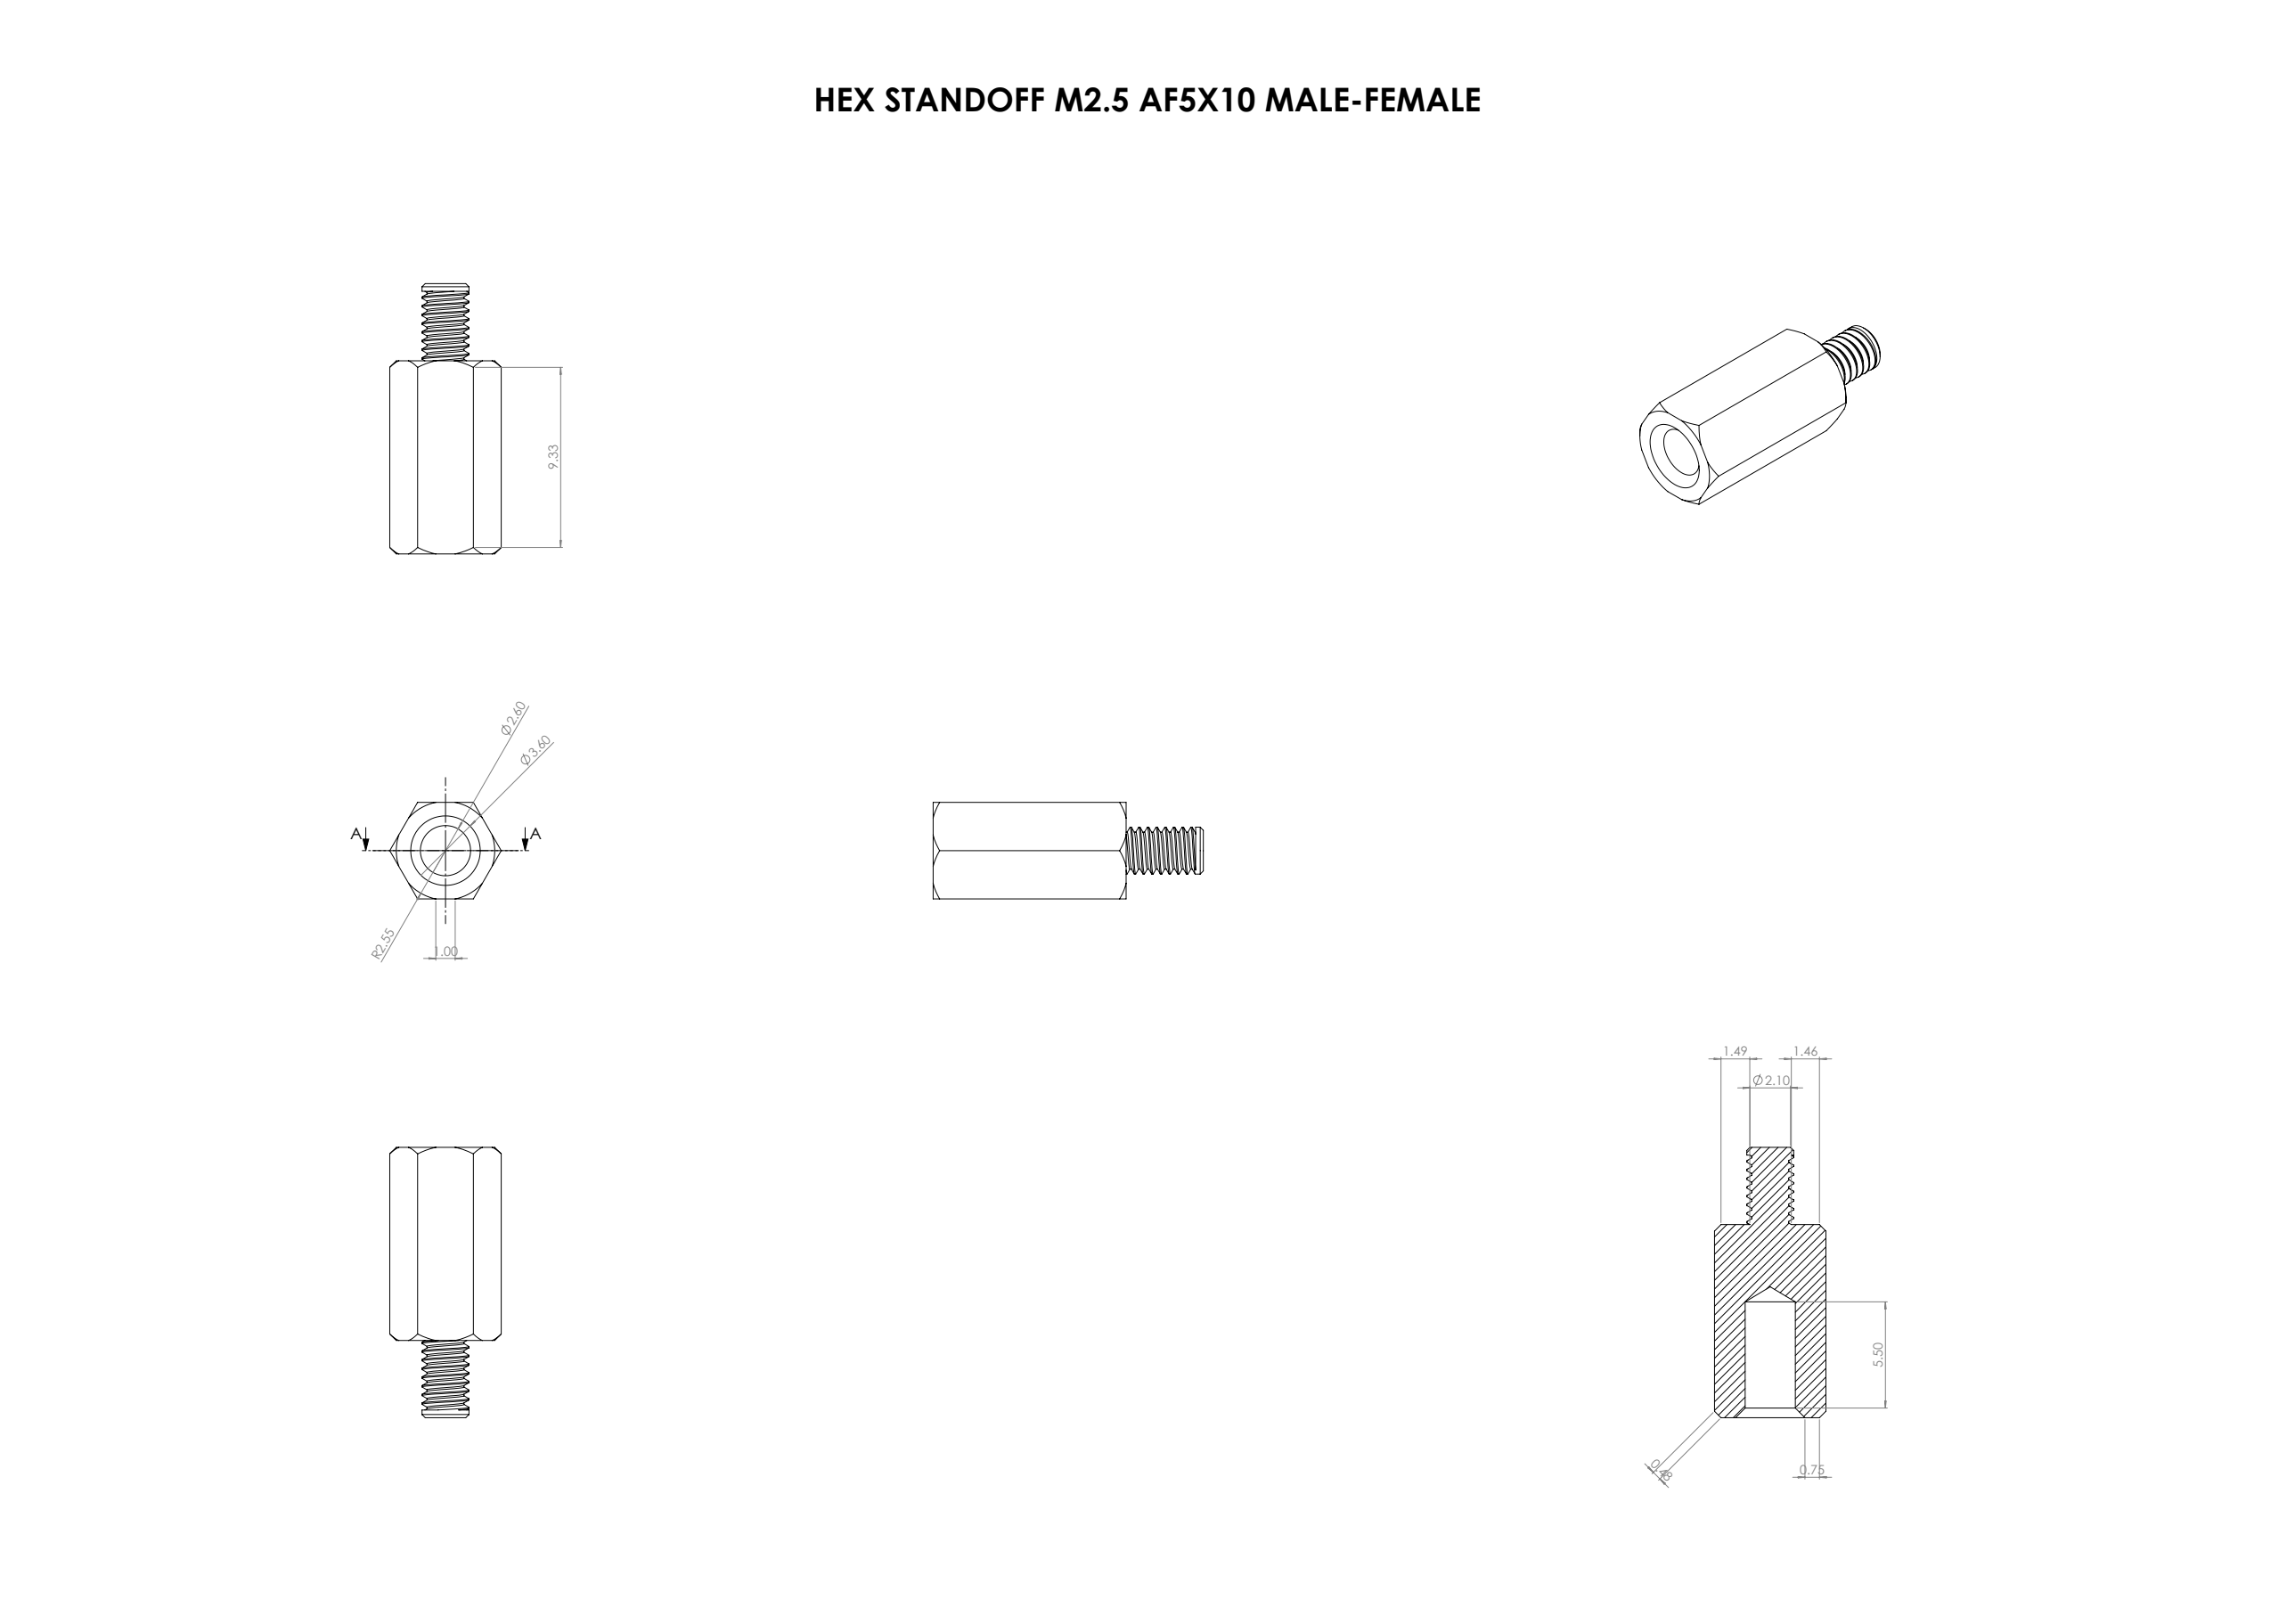
ISO-10303-21;
HEADER;
/* Generated by software containing ST-Developer
 * from STEP Tools, Inc. (www.steptools.com) 
 */

FILE_DESCRIPTION(
/* description */ (''),
/* implementation_level */ '2;1');

FILE_NAME(
/* name */ '14_Hex_Standoff_M2.5_AF5x10_Male-Female.step',
/* time_stamp */ '2026-10-19T23:00:43-07:00',
/* author */ (''),
/* organization */ (''),
/* preprocessor_version */ 'ST-DEVELOPER v20.2',
/* originating_system */ 'Autodesk Translation Framework v15.15.0.0',
/* authorisation */ '');

FILE_SCHEMA (('AUTOMOTIVE_DESIGN { 1 0 10303 214 3 1 1 }'));
ENDSEC;

DATA;
#10=MECHANICAL_DESIGN_GEOMETRIC_PRESENTATION_REPRESENTATION('',(#1010),#55002);
#227=(
BOUNDED_CURVE()
B_SPLINE_CURVE(2,(#39814,#39815,#39816),.UNSPECIFIED.,.F.,.F.)
B_SPLINE_CURVE_WITH_KNOTS((3,3),(0.0560176289802603,0.163687850794567),
 .UNSPECIFIED.)
CURVE()
GEOMETRIC_REPRESENTATION_ITEM()
RATIONAL_B_SPLINE_CURVE((1.01603499393247,1.02342774714042,1.))
REPRESENTATION_ITEM('')
);
#228=(
BOUNDED_CURVE()
B_SPLINE_CURVE(2,(#39818,#39819,#39820),.UNSPECIFIED.,.F.,.F.)
B_SPLINE_CURVE_WITH_KNOTS((3,3),(0.,0.107670221814307),.UNSPECIFIED.)
CURVE()
GEOMETRIC_REPRESENTATION_ITEM()
RATIONAL_B_SPLINE_CURVE((1.,1.02342774714043,1.01603499393248))
REPRESENTATION_ITEM('')
);
#229=(
BOUNDED_CURVE()
B_SPLINE_CURVE(2,(#39825,#39826,#39827),.UNSPECIFIED.,.F.,.F.)
B_SPLINE_CURVE_WITH_KNOTS((3,3),(0.0560176289802603,0.163687850794567),
 .UNSPECIFIED.)
CURVE()
GEOMETRIC_REPRESENTATION_ITEM()
RATIONAL_B_SPLINE_CURVE((1.01603499393248,1.02342774714042,1.))
REPRESENTATION_ITEM('')
);
#230=(
BOUNDED_CURVE()
B_SPLINE_CURVE(2,(#39829,#39830,#39831),.UNSPECIFIED.,.F.,.F.)
B_SPLINE_CURVE_WITH_KNOTS((3,3),(0.,0.107670221814307),.UNSPECIFIED.)
CURVE()
GEOMETRIC_REPRESENTATION_ITEM()
RATIONAL_B_SPLINE_CURVE((1.,1.02342774714042,1.01603499393248))
REPRESENTATION_ITEM('')
);
#231=(
BOUNDED_CURVE()
B_SPLINE_CURVE(2,(#39836,#39837,#39838),.UNSPECIFIED.,.F.,.F.)
B_SPLINE_CURVE_WITH_KNOTS((3,3),(0.0560176289802603,0.163687850794567),
 .UNSPECIFIED.)
CURVE()
GEOMETRIC_REPRESENTATION_ITEM()
RATIONAL_B_SPLINE_CURVE((1.01603499393248,1.02342774714042,1.))
REPRESENTATION_ITEM('')
);
#232=(
BOUNDED_CURVE()
B_SPLINE_CURVE(2,(#39840,#39841,#39842),.UNSPECIFIED.,.F.,.F.)
B_SPLINE_CURVE_WITH_KNOTS((3,3),(0.,0.107670221814307),.UNSPECIFIED.)
CURVE()
GEOMETRIC_REPRESENTATION_ITEM()
RATIONAL_B_SPLINE_CURVE((1.,1.02342774714043,1.01603499393248))
REPRESENTATION_ITEM('')
);
#233=(
BOUNDED_CURVE()
B_SPLINE_CURVE(2,(#39847,#39848,#39849),.UNSPECIFIED.,.F.,.F.)
B_SPLINE_CURVE_WITH_KNOTS((3,3),(0.0560176289802605,0.163687850794567),
 .UNSPECIFIED.)
CURVE()
GEOMETRIC_REPRESENTATION_ITEM()
RATIONAL_B_SPLINE_CURVE((1.01603499393247,1.02342774714041,1.))
REPRESENTATION_ITEM('')
);
#234=(
BOUNDED_CURVE()
B_SPLINE_CURVE(2,(#39851,#39852,#39853),.UNSPECIFIED.,.F.,.F.)
B_SPLINE_CURVE_WITH_KNOTS((3,3),(0.,0.107670221814307),.UNSPECIFIED.)
CURVE()
GEOMETRIC_REPRESENTATION_ITEM()
RATIONAL_B_SPLINE_CURVE((1.,1.02342774714042,1.01603499393247))
REPRESENTATION_ITEM('')
);
#235=(
BOUNDED_CURVE()
B_SPLINE_CURVE(2,(#39858,#39859,#39860),.UNSPECIFIED.,.F.,.F.)
B_SPLINE_CURVE_WITH_KNOTS((3,3),(0.0560176289802603,0.163687850794567),
 .UNSPECIFIED.)
CURVE()
GEOMETRIC_REPRESENTATION_ITEM()
RATIONAL_B_SPLINE_CURVE((1.01603499393247,1.02342774714041,1.))
REPRESENTATION_ITEM('')
);
#236=(
BOUNDED_CURVE()
B_SPLINE_CURVE(2,(#39862,#39863,#39864),.UNSPECIFIED.,.F.,.F.)
B_SPLINE_CURVE_WITH_KNOTS((3,3),(0.,0.107670221814307),.UNSPECIFIED.)
CURVE()
GEOMETRIC_REPRESENTATION_ITEM()
RATIONAL_B_SPLINE_CURVE((1.,1.02342774714042,1.01603499393247))
REPRESENTATION_ITEM('')
);
#237=(
BOUNDED_CURVE()
B_SPLINE_CURVE(2,(#39869,#39870,#39871),.UNSPECIFIED.,.F.,.F.)
B_SPLINE_CURVE_WITH_KNOTS((3,3),(0.,0.107670221814307),.UNSPECIFIED.)
CURVE()
GEOMETRIC_REPRESENTATION_ITEM()
RATIONAL_B_SPLINE_CURVE((1.,1.02342774714043,1.01603499393248))
REPRESENTATION_ITEM('')
);
#238=(
BOUNDED_CURVE()
B_SPLINE_CURVE(2,(#39874,#39875,#39876),.UNSPECIFIED.,.F.,.F.)
B_SPLINE_CURVE_WITH_KNOTS((3,3),(0.0560176289802603,0.163687850794567),
 .UNSPECIFIED.)
CURVE()
GEOMETRIC_REPRESENTATION_ITEM()
RATIONAL_B_SPLINE_CURVE((1.01603499393247,1.02342774714042,1.))
REPRESENTATION_ITEM('')
);
#239=(
BOUNDED_CURVE()
B_SPLINE_CURVE(2,(#39881,#39882,#39883),.UNSPECIFIED.,.F.,.F.)
B_SPLINE_CURVE_WITH_KNOTS((3,3),(0.0560176289802605,0.163687850794567),
 .UNSPECIFIED.)
CURVE()
GEOMETRIC_REPRESENTATION_ITEM()
RATIONAL_B_SPLINE_CURVE((1.01603499393247,1.02342774714041,1.))
REPRESENTATION_ITEM('')
);
#240=(
BOUNDED_CURVE()
B_SPLINE_CURVE(2,(#39887,#39888,#39889),.UNSPECIFIED.,.F.,.F.)
B_SPLINE_CURVE_WITH_KNOTS((3,3),(0.,0.107670221814307),.UNSPECIFIED.)
CURVE()
GEOMETRIC_REPRESENTATION_ITEM()
RATIONAL_B_SPLINE_CURVE((1.,1.02342774714041,1.01603499393247))
REPRESENTATION_ITEM('')
);
#241=(
BOUNDED_CURVE()
B_SPLINE_CURVE(2,(#39894,#39895,#39896),.UNSPECIFIED.,.F.,.F.)
B_SPLINE_CURVE_WITH_KNOTS((3,3),(0.0560176289802601,0.163687850794567),
 .UNSPECIFIED.)
CURVE()
GEOMETRIC_REPRESENTATION_ITEM()
RATIONAL_B_SPLINE_CURVE((1.01603499393247,1.02342774714041,1.))
REPRESENTATION_ITEM('')
);
#242=(
BOUNDED_CURVE()
B_SPLINE_CURVE(2,(#39900,#39901,#39902),.UNSPECIFIED.,.F.,.F.)
B_SPLINE_CURVE_WITH_KNOTS((3,3),(0.,0.107670221814307),.UNSPECIFIED.)
CURVE()
GEOMETRIC_REPRESENTATION_ITEM()
RATIONAL_B_SPLINE_CURVE((1.,1.02342774714041,1.01603499393247))
REPRESENTATION_ITEM('')
);
#243=(
BOUNDED_CURVE()
B_SPLINE_CURVE(2,(#39907,#39908,#39909),.UNSPECIFIED.,.F.,.F.)
B_SPLINE_CURVE_WITH_KNOTS((3,3),(0.0560176289802598,0.163687850794567),
 .UNSPECIFIED.)
CURVE()
GEOMETRIC_REPRESENTATION_ITEM()
RATIONAL_B_SPLINE_CURVE((1.01603499393248,1.02342774714042,1.))
REPRESENTATION_ITEM('')
);
#244=(
BOUNDED_CURVE()
B_SPLINE_CURVE(2,(#39913,#39914,#39915),.UNSPECIFIED.,.F.,.F.)
B_SPLINE_CURVE_WITH_KNOTS((3,3),(0.,0.107670221814307),.UNSPECIFIED.)
CURVE()
GEOMETRIC_REPRESENTATION_ITEM()
RATIONAL_B_SPLINE_CURVE((1.,1.02342774714041,1.01603499393247))
REPRESENTATION_ITEM('')
);
#245=(
BOUNDED_CURVE()
B_SPLINE_CURVE(2,(#39924,#39925,#39926),.UNSPECIFIED.,.F.,.F.)
B_SPLINE_CURVE_WITH_KNOTS((3,3),(0.0560176289802602,0.163687850794567),
 .UNSPECIFIED.)
CURVE()
GEOMETRIC_REPRESENTATION_ITEM()
RATIONAL_B_SPLINE_CURVE((1.01603499393248,1.02342774714042,1.))
REPRESENTATION_ITEM('')
);
#246=(
BOUNDED_CURVE()
B_SPLINE_CURVE(2,(#39930,#39931,#39932),.UNSPECIFIED.,.F.,.F.)
B_SPLINE_CURVE_WITH_KNOTS((3,3),(0.,0.107670221814307),.UNSPECIFIED.)
CURVE()
GEOMETRIC_REPRESENTATION_ITEM()
RATIONAL_B_SPLINE_CURVE((1.,1.02342774714041,1.01603499393247))
REPRESENTATION_ITEM('')
);
#247=(
BOUNDED_CURVE()
B_SPLINE_CURVE(2,(#39937,#39938,#39939),.UNSPECIFIED.,.F.,.F.)
B_SPLINE_CURVE_WITH_KNOTS((3,3),(0.,0.107670221814307),.UNSPECIFIED.)
CURVE()
GEOMETRIC_REPRESENTATION_ITEM()
RATIONAL_B_SPLINE_CURVE((1.,1.02342774714041,1.01603499393247))
REPRESENTATION_ITEM('')
);
#248=(
BOUNDED_CURVE()
B_SPLINE_CURVE(2,(#39942,#39943,#39944),.UNSPECIFIED.,.F.,.F.)
B_SPLINE_CURVE_WITH_KNOTS((3,3),(0.0560176289802595,0.163687850794568),
 .UNSPECIFIED.)
CURVE()
GEOMETRIC_REPRESENTATION_ITEM()
RATIONAL_B_SPLINE_CURVE((1.01603499393248,1.02342774714043,1.))
REPRESENTATION_ITEM('')
);
#249=(
BOUNDED_CURVE()
B_SPLINE_CURVE(2,(#39948,#39949,#39950),.UNSPECIFIED.,.F.,.F.)
B_SPLINE_CURVE_WITH_KNOTS((3,3),(0.05601762898026,0.163687850794567),
 .UNSPECIFIED.)
CURVE()
GEOMETRIC_REPRESENTATION_ITEM()
RATIONAL_B_SPLINE_CURVE((1.01603499393247,1.02342774714041,1.))
REPRESENTATION_ITEM('')
);
#250=(
BOUNDED_CURVE()
B_SPLINE_CURVE(2,(#39959,#39960,#39961),.UNSPECIFIED.,.F.,.F.)
B_SPLINE_CURVE_WITH_KNOTS((3,3),(0.,0.107670221814308),.UNSPECIFIED.)
CURVE()
GEOMETRIC_REPRESENTATION_ITEM()
RATIONAL_B_SPLINE_CURVE((1.,1.02342774714044,1.01603499393249))
REPRESENTATION_ITEM('')
);
#472=B_SPLINE_SURFACE_WITH_KNOTS('',3,3,((#39118,#39119,#39120,#39121,#39122,
#39123,#39124,#39125,#39126,#39127,#39128,#39129,#39130,#39131,#39132,#39133,
#39134,#39135,#39136,#39137,#39138,#39139,#39140,#39141,#39142,#39143,#39144,
#39145,#39146,#39147,#39148,#39149,#39150,#39151,#39152,#39153,#39154,#39155,
#39156,#39157,#39158,#39159,#39160,#39161,#39162,#39163,#39164,#39165,#39166,
#39167,#39168,#39169,#39170,#39171,#39172,#39173),(#39174,#39175,#39176,
#39177,#39178,#39179,#39180,#39181,#39182,#39183,#39184,#39185,#39186,#39187,
#39188,#39189,#39190,#39191,#39192,#39193,#39194,#39195,#39196,#39197,#39198,
#39199,#39200,#39201,#39202,#39203,#39204,#39205,#39206,#39207,#39208,#39209,
#39210,#39211,#39212,#39213,#39214,#39215,#39216,#39217,#39218,#39219,#39220,
#39221,#39222,#39223,#39224,#39225,#39226,#39227,#39228,#39229),(#39230,
#39231,#39232,#39233,#39234,#39235,#39236,#39237,#39238,#39239,#39240,#39241,
#39242,#39243,#39244,#39245,#39246,#39247,#39248,#39249,#39250,#39251,#39252,
#39253,#39254,#39255,#39256,#39257,#39258,#39259,#39260,#39261,#39262,#39263,
#39264,#39265,#39266,#39267,#39268,#39269,#39270,#39271,#39272,#39273,#39274,
#39275,#39276,#39277,#39278,#39279,#39280,#39281,#39282,#39283,#39284,#39285),
(#39286,#39287,#39288,#39289,#39290,#39291,#39292,#39293,#39294,#39295,
#39296,#39297,#39298,#39299,#39300,#39301,#39302,#39303,#39304,#39305,#39306,
#39307,#39308,#39309,#39310,#39311,#39312,#39313,#39314,#39315,#39316,#39317,
#39318,#39319,#39320,#39321,#39322,#39323,#39324,#39325,#39326,#39327,#39328,
#39329,#39330,#39331,#39332,#39333,#39334,#39335,#39336,#39337,#39338,#39339,
#39340,#39341)),.UNSPECIFIED.,.F.,.F.,.F.,(4,4),(4,1,1,1,1,1,1,1,1,1,1,
1,1,1,1,1,1,1,1,1,1,1,1,1,1,1,1,1,1,1,1,1,1,1,1,1,1,1,1,1,1,1,1,1,1,1,1,
1,1,1,1,1,1,4),(0.,0.0296469363228873),(11.5874873465742,12.5749444987495,
13.5624016509248,14.5498588031001,15.5373159552754,16.5247731074507,17.512230259626,
18.4996874118013,19.4871445639766,20.4746017161519,21.4620588683272,22.4495160205025,
23.4369731726778,24.4244303248531,25.4118874770284,26.3993446292037,27.386801781379,
28.3742589335543,29.3617160857296,30.3491732379048,31.3366303900801,32.3240875422554,
33.3115446944307,34.299001846606,35.2864589987813,36.2739161509566,37.2613733031319,
38.2488304553072,39.2362876074825,40.2237447596578,41.2112019118331,42.1986590640084,
43.1861162161837,44.173573368359,45.1610305205343,46.1484876727096,47.1359448248849,
48.1234019770602,49.1108591292355,50.0983162814107,51.085773433586,52.0732305857613,
53.0606877379366,54.0481448901119,55.0356020422872,56.0230591944625,57.0105163466378,
57.9979734988131,58.9854306509884,59.9728878031637,60.960344955339,61.9478021075143,
62.9352592596896,63.9227164118649),.UNSPECIFIED.);
#473=B_SPLINE_SURFACE_WITH_KNOTS('',3,3,((#39515,#39516,#39517,#39518,#39519,
#39520,#39521,#39522,#39523,#39524,#39525,#39526,#39527,#39528,#39529,#39530,
#39531,#39532,#39533,#39534,#39535,#39536,#39537,#39538,#39539,#39540,#39541,
#39542,#39543,#39544,#39545,#39546,#39547,#39548,#39549,#39550,#39551,#39552,
#39553,#39554,#39555,#39556,#39557,#39558,#39559,#39560,#39561,#39562,#39563,
#39564,#39565,#39566,#39567,#39568,#39569,#39570),(#39571,#39572,#39573,
#39574,#39575,#39576,#39577,#39578,#39579,#39580,#39581,#39582,#39583,#39584,
#39585,#39586,#39587,#39588,#39589,#39590,#39591,#39592,#39593,#39594,#39595,
#39596,#39597,#39598,#39599,#39600,#39601,#39602,#39603,#39604,#39605,#39606,
#39607,#39608,#39609,#39610,#39611,#39612,#39613,#39614,#39615,#39616,#39617,
#39618,#39619,#39620,#39621,#39622,#39623,#39624,#39625,#39626),(#39627,
#39628,#39629,#39630,#39631,#39632,#39633,#39634,#39635,#39636,#39637,#39638,
#39639,#39640,#39641,#39642,#39643,#39644,#39645,#39646,#39647,#39648,#39649,
#39650,#39651,#39652,#39653,#39654,#39655,#39656,#39657,#39658,#39659,#39660,
#39661,#39662,#39663,#39664,#39665,#39666,#39667,#39668,#39669,#39670,#39671,
#39672,#39673,#39674,#39675,#39676,#39677,#39678,#39679,#39680,#39681,#39682),
(#39683,#39684,#39685,#39686,#39687,#39688,#39689,#39690,#39691,#39692,
#39693,#39694,#39695,#39696,#39697,#39698,#39699,#39700,#39701,#39702,#39703,
#39704,#39705,#39706,#39707,#39708,#39709,#39710,#39711,#39712,#39713,#39714,
#39715,#39716,#39717,#39718,#39719,#39720,#39721,#39722,#39723,#39724,#39725,
#39726,#39727,#39728,#39729,#39730,#39731,#39732,#39733,#39734,#39735,#39736,
#39737,#39738)),.UNSPECIFIED.,.F.,.F.,.F.,(4,4),(4,1,1,1,1,1,1,1,1,1,1,
1,1,1,1,1,1,1,1,1,1,1,1,1,1,1,1,1,1,1,1,1,1,1,1,1,1,1,1,1,1,1,1,1,1,1,1,
1,1,1,1,1,1,4),(0.,0.0296469363228873),(14.896352608199,15.8838097603743,
16.8712669125496,17.8587240647249,18.8461812169001,19.8336383690754,20.8210955212507,
21.808552673426,22.7960098256013,23.7834669777766,24.7709241299519,25.7583812821272,
26.7458384343025,27.7332955864778,28.7207527386531,29.7082098908284,30.6956670430037,
31.683124195179,32.6705813473543,33.6580384995296,34.6454956517049,35.6329528038802,
36.6204099560555,37.6078671082307,38.595324260406,39.5827814125813,40.5702385647566,
41.5576957169319,42.5451528691072,43.5326100212825,44.5200671734578,45.5075243256331,
46.4949814778084,47.4824386299837,48.469895782159,49.4573529343343,50.4448100865096,
51.4322672386849,52.4197243908602,53.4071815430355,54.3946386952108,55.3820958473861,
56.3695529995614,57.3570101517367,58.3444673039119,59.3319244560872,60.3193816082625,
61.3068387604378,62.2942959126131,63.2817530647884,64.2692102169637,65.256667369139,
66.2441245213143,67.2315816734896),.UNSPECIFIED.);
#528=B_SPLINE_CURVE_WITH_KNOTS('',3,(#38534,#38535,#38536,#38537,#38538,
#38539,#38540,#38541,#38542,#38543,#38544,#38545,#38546,#38547,#38548,#38549,
#38550,#38551,#38552),.UNSPECIFIED.,.F.,.F.,(4,3,3,3,3,3,4),(-7.09479596692956,
-6.91220006522707,-5.92474291305177,-4.93728576087648,-3.94982860870118,
-2.96237145652589,-2.06974660785394),.UNSPECIFIED.);
#529=B_SPLINE_CURVE_WITH_KNOTS('',3,(#38560,#38561,#38562,#38563,#38564,
#38565,#38566,#38567,#38568,#38569,#38570,#38571,#38572,#38573,#38574,#38575),
 .UNSPECIFIED.,.F.,.F.,(4,3,3,3,3,4),(0.,0.987457152175289,1.97491430435059,
2.96237145652588,3.94982860870118,4.12047592137467),.UNSPECIFIED.);
#530=B_SPLINE_CURVE_WITH_KNOTS('',3,(#38580,#38581,#38582,#38583,#38584,
#38585,#38586,#38587,#38588,#38589,#38590,#38591,#38592,#38593,#38594,#38595,
#38596,#38597,#38598,#38599,#38600,#38601),.UNSPECIFIED.,.F.,.F.,(4,3,3,
3,3,3,3,4),(-13.3779812741091,-12.8369429782788,-11.8494858261035,-10.8620286739282,
-9.87457152175295,-8.88711436957765,-7.89965721740236,-7.09479596692956),
 .UNSPECIFIED.);
#531=B_SPLINE_CURVE_WITH_KNOTS('',3,(#38602,#38603,#38604,#38605,#38606,
#38607,#38608,#38609,#38610,#38611,#38612,#38613,#38614,#38615,#38616,#38617,
#38618,#38619,#38620,#38621,#38622,#38623),.UNSPECIFIED.,.F.,.F.,(4,3,3,
3,3,3,3,4),(4.12047592137467,4.93728576087648,5.92474291305177,6.91220006522707,
7.89965721740236,8.88711436957765,9.87457152175295,10.4036612285542),
 .UNSPECIFIED.);
#532=B_SPLINE_CURVE_WITH_KNOTS('',3,(#38628,#38629,#38630,#38631,#38632,
#38633,#38634,#38635,#38636,#38637,#38638,#38639,#38640,#38641,#38642,#38643,
#38644,#38645,#38646,#38647,#38648,#38649),.UNSPECIFIED.,.F.,.F.,(4,3,3,
3,3,3,3,4),(-19.6611665812887,-18.7616858913306,-17.7742287391553,-16.78677158698,
-15.7993144348047,-14.8118572826294,-13.8244001304541,-13.3779812741091),
 .UNSPECIFIED.);
#533=B_SPLINE_CURVE_WITH_KNOTS('',3,(#38650,#38651,#38652,#38653,#38654,
#38655,#38656,#38657,#38658,#38659,#38660,#38661,#38662,#38663,#38664,#38665,
#38666,#38667,#38668,#38669,#38670,#38671),.UNSPECIFIED.,.F.,.F.,(4,3,3,
3,3,3,3,4),(10.4036612285542,10.8620286739282,11.8494858261035,12.8369429782788,
13.8244001304541,14.8118572826294,15.7993144348047,16.6868465357338),
 .UNSPECIFIED.);
#534=B_SPLINE_CURVE_WITH_KNOTS('',3,(#38676,#38677,#38678,#38679,#38680,
#38681,#38682,#38683,#38684,#38685,#38686,#38687,#38688,#38689,#38690,#38691,
#38692,#38693,#38694,#38695,#38696,#38697,#38698,#38699,#38700),
 .UNSPECIFIED.,.F.,.F.,(4,3,3,3,3,3,3,3,4),(-25.9443518884683,-25.6738859565577,
-24.6864288043824,-23.6989716522071,-22.7115145000318,-21.7240573478565,
-20.7366001956812,-19.7491430435059,-19.6611665812887),.UNSPECIFIED.);
#535=B_SPLINE_CURVE_WITH_KNOTS('',3,(#38701,#38702,#38703,#38704,#38705,
#38706,#38707,#38708,#38709,#38710,#38711,#38712,#38713,#38714,#38715,#38716,
#38717,#38718,#38719,#38720,#38721,#38722,#38723,#38724,#38725),
 .UNSPECIFIED.,.F.,.F.,(4,3,3,3,3,3,3,3,4),(16.6868465357338,16.78677158698,
17.7742287391553,18.7616858913306,19.7491430435059,20.7366001956812,21.7240573478565,
22.7115145000318,22.9700318429134),.UNSPECIFIED.);
#536=B_SPLINE_CURVE_WITH_KNOTS('',3,(#38730,#38731,#38732,#38733,#38734,
#38735,#38736,#38737,#38738,#38739,#38740,#38741,#38742,#38743,#38744,#38745,
#38746,#38747,#38748,#38749,#38750,#38751),.UNSPECIFIED.,.F.,.F.,(4,3,3,
3,3,3,3,4),(-32.2275371956479,-31.5986288696094,-30.6111717174341,-29.6237145652589,
-28.6362574130836,-27.6488002609083,-26.661343108733,-25.9443518884683),
 .UNSPECIFIED.);
#537=B_SPLINE_CURVE_WITH_KNOTS('',3,(#38752,#38753,#38754,#38755,#38756,
#38757,#38758,#38759,#38760,#38761,#38762,#38763,#38764,#38765,#38766,#38767,
#38768,#38769,#38770,#38771,#38772,#38773),.UNSPECIFIED.,.F.,.F.,(4,3,3,
3,3,3,3,4),(22.9700318429134,23.6989716522071,24.6864288043824,25.6738859565577,
26.661343108733,27.6488002609083,28.6362574130836,29.253217150093),
 .UNSPECIFIED.);
#538=B_SPLINE_CURVE_WITH_KNOTS('',3,(#38778,#38779,#38780,#38781,#38782,
#38783,#38784,#38785,#38786,#38787,#38788,#38789,#38790,#38791,#38792,#38793,
#38794,#38795,#38796,#38797,#38798,#38799),.UNSPECIFIED.,.F.,.F.,(4,3,3,
3,3,3,3,4),(-38.5107225028275,-37.5233717826612,-36.5359146304859,-35.5484574783106,
-34.5610003261353,-33.57354317396,-32.5860860217847,-32.2275371956479),
 .UNSPECIFIED.);
#539=B_SPLINE_CURVE_WITH_KNOTS('',3,(#38800,#38801,#38802,#38803,#38804,
#38805,#38806,#38807,#38808,#38809,#38810,#38811,#38812,#38813,#38814,#38815,
#38816,#38817,#38818,#38819,#38820,#38821),.UNSPECIFIED.,.F.,.F.,(4,3,3,
3,3,3,3,4),(29.253217150093,29.6237145652588,30.6111717174341,31.5986288696094,
32.5860860217847,33.57354317396,34.5610003261353,35.5364024572726),
 .UNSPECIFIED.);
#540=B_SPLINE_CURVE_WITH_KNOTS('',3,(#38826,#38827,#38828,#38829,#38830,
#38831,#38832,#38833,#38834,#38835,#38836,#38837,#38838,#38839,#38840,#38841,
#38842,#38843,#38844,#38845,#38846,#38847),.UNSPECIFIED.,.F.,.F.,(4,3,3,
3,3,3,3,4),(-44.7939078100071,-44.4355718478883,-43.448114695713,-42.4606575435377,
-41.4732003913624,-40.4857432391871,-39.4982860870118,-38.5107225028275),
 .UNSPECIFIED.);
#541=B_SPLINE_CURVE_WITH_KNOTS('',3,(#38848,#38849,#38850,#38851,#38852,
#38853,#38854,#38855,#38856,#38857,#38858,#38859,#38860,#38861,#38862,#38863,
#38864,#38865,#38866,#38867,#38868,#38869,#38870,#38871,#38872),
 .UNSPECIFIED.,.F.,.F.,(4,3,3,3,3,3,3,3,4),(35.5364024572726,35.5484574783106,
36.5359146304859,37.5233717826612,38.5108289348365,39.4982860870118,40.4857432391871,
41.4732003913624,41.8195877644522),.UNSPECIFIED.);
#542=B_SPLINE_CURVE_WITH_KNOTS('',3,(#38877,#38878,#38879,#38880,#38881,
#38882,#38883,#38884,#38885,#38886,#38887,#38888,#38889,#38890,#38891,#38892,
#38893,#38894,#38895,#38896,#38897,#38898),.UNSPECIFIED.,.F.,.F.,(4,3,3,
3,3,3,3,4),(-51.0770931171867,-50.36031476094,-49.3728576087648,-48.3854004565895,
-47.3979433044142,-46.4104861522389,-45.4230290000636,-44.7939078100071),
 .UNSPECIFIED.);
#543=B_SPLINE_CURVE_WITH_KNOTS('',3,(#38899,#38900,#38901,#38902,#38903,
#38904,#38905,#38906,#38907,#38908,#38909,#38910,#38911,#38912,#38913,#38914,
#38915,#38916,#38917,#38918,#38919,#38920),.UNSPECIFIED.,.F.,.F.,(4,3,3,
3,3,3,3,4),(41.8195877644522,42.4606575435377,43.448114695713,44.4355718478883,
45.4230290000636,46.4104861522389,47.3979433044142,48.1027730716318),
 .UNSPECIFIED.);
#544=B_SPLINE_CURVE_WITH_KNOTS('',3,(#38926,#38927,#38928,#38929,#38930,
#38931,#38932,#38933,#38934),.UNSPECIFIED.,.F.,.F.,(4,1,1,1,1,1,4),(59.6902604182061,
60.3193816082625,61.3068387604378,62.2942959126131,63.2817530647884,64.2692102169637,
65.1618350656357),.UNSPECIFIED.);
#545=B_SPLINE_CURVE_WITH_KNOTS('',3,(#38937,#38938,#38939,#38940,#38941,
#38942,#38943,#38944),.UNSPECIFIED.,.F.,.F.,(4,1,1,1,1,4),(59.6902604182061,
59.9728878031637,60.960344955339,61.9478021075143,62.9352592596896,63.9227164118649),
 .UNSPECIFIED.);
#546=B_SPLINE_CURVE_WITH_KNOTS('',3,(#38949,#38950,#38951,#38952,#38953,
#38954,#38955,#38956,#38957,#38958,#38959),.UNSPECIFIED.,.F.,.F.,(4,1,1,
1,1,1,1,1,4),(53.4070751110265,53.4071815430355,54.3946386952108,55.3820958473861,
56.3695529995614,57.3570101517367,58.3444673039119,59.3319244560872,59.6902604182061),
 .UNSPECIFIED.);
#547=B_SPLINE_CURVE_WITH_KNOTS('',3,(#38960,#38961,#38962,#38963,#38964,
#38965,#38966,#38967,#38968,#38969),.UNSPECIFIED.,.F.,.F.,(4,1,1,1,1,1,
1,4),(53.4070751110265,54.0481448901119,55.0356020422872,56.0230591944625,
57.0105163466378,57.9979734988131,58.9854306509884,59.6902604182061),
 .UNSPECIFIED.);
#548=B_SPLINE_CURVE_WITH_KNOTS('',3,(#38974,#38975,#38976,#38977,#38978,
#38979,#38980,#38981,#38982,#38983),.UNSPECIFIED.,.F.,.F.,(4,1,1,1,1,1,
1,4),(47.1238898038469,47.4824386299837,48.469895782159,49.4573529343343,
50.4448100865096,51.4322672386849,52.4197243908602,53.4070751110265),
 .UNSPECIFIED.);
#549=B_SPLINE_CURVE_WITH_KNOTS('',3,(#38984,#38985,#38986,#38987,#38988,
#38989,#38990,#38991,#38992,#38993,#38994),.UNSPECIFIED.,.F.,.F.,(4,1,1,
1,1,1,1,1,4),(47.1238898038469,47.1359448248849,48.1234019770602,49.1108591292355,
50.0983162814107,51.085773433586,52.0732305857613,53.0606877379366,53.4070751110265),
 .UNSPECIFIED.);
#550=B_SPLINE_CURVE_WITH_KNOTS('',3,(#38999,#39000,#39001,#39002,#39003,
#39004,#39005,#39006,#39007,#39008),.UNSPECIFIED.,.F.,.F.,(4,1,1,1,1,1,
1,4),(40.8407044966673,41.5576957169319,42.5451528691072,43.5326100212825,
44.5200671734578,45.5075243256331,46.4949814778084,47.1238898038469),
 .UNSPECIFIED.);
#551=B_SPLINE_CURVE_WITH_KNOTS('',3,(#39009,#39010,#39011,#39012,#39013,
#39014,#39015,#39016,#39017,#39018),.UNSPECIFIED.,.F.,.F.,(4,1,1,1,1,1,
1,4),(40.8407044966673,41.2112019118331,42.1986590640084,43.1861162161837,
44.173573368359,45.1610305205343,46.1484876727096,47.1238898038469),
 .UNSPECIFIED.);
#552=B_SPLINE_CURVE_WITH_KNOTS('',3,(#39023,#39024,#39025,#39026,#39027,
#39028,#39029,#39030,#39031,#39032,#39033),.UNSPECIFIED.,.F.,.F.,(4,1,1,
1,1,1,1,1,4),(34.5575191894877,34.6454956517049,35.6329528038802,36.6204099560555,
37.6078671082307,38.595324260406,39.5827814125813,40.5702385647566,40.8407044966673),
 .UNSPECIFIED.);
#553=B_SPLINE_CURVE_WITH_KNOTS('',3,(#39034,#39035,#39036,#39037,#39038,
#39039,#39040,#39041,#39042,#39043),.UNSPECIFIED.,.F.,.F.,(4,1,1,1,1,1,
1,4),(34.5575191894877,35.2864589987813,36.2739161509566,37.2613733031319,
38.2488304553072,39.2362876074825,40.2237447596578,40.8407044966673),
 .UNSPECIFIED.);
#554=B_SPLINE_CURVE_WITH_KNOTS('',3,(#39048,#39049,#39050,#39051,#39052,
#39053,#39054,#39055,#39056,#39057),.UNSPECIFIED.,.F.,.F.,(4,1,1,1,1,1,
1,4),(28.2743338823081,28.7207527386531,29.7082098908284,30.6956670430037,
31.683124195179,32.6705813473543,33.6580384995296,34.5575191894877),
 .UNSPECIFIED.);
#555=B_SPLINE_CURVE_WITH_KNOTS('',3,(#39058,#39059,#39060,#39061,#39062,
#39063,#39064,#39065,#39066,#39067,#39068),.UNSPECIFIED.,.F.,.F.,(4,1,1,
1,1,1,1,1,4),(28.2743338823081,28.3742589335543,29.3617160857296,30.3491732379048,
31.3366303900801,32.3240875422554,33.3115446944307,34.299001846606,34.5575191894877),
 .UNSPECIFIED.);
#556=B_SPLINE_CURVE_WITH_KNOTS('',3,(#39073,#39074,#39075,#39076,#39077,
#39078,#39079,#39080,#39081,#39082),.UNSPECIFIED.,.F.,.F.,(4,1,1,1,1,1,
1,4),(21.9911485751285,22.7960098256013,23.7834669777766,24.7709241299519,
25.7583812821272,26.7458384343025,27.7332955864778,28.2743338823081),
 .UNSPECIFIED.);
#557=B_SPLINE_CURVE_WITH_KNOTS('',3,(#39083,#39084,#39085,#39086,#39087,
#39088,#39089,#39090,#39091,#39092),.UNSPECIFIED.,.F.,.F.,(4,1,1,1,1,1,
1,4),(21.9911485751285,22.4495160205025,23.4369731726778,24.4244303248531,
25.4118874770284,26.3993446292037,27.386801781379,28.2743338823081),
 .UNSPECIFIED.);
#558=B_SPLINE_CURVE_WITH_KNOTS('',3,(#39097,#39098,#39099,#39100,#39101,
#39102,#39103,#39104,#39105,#39106,#39107),.UNSPECIFIED.,.F.,.F.,(4,1,1,
1,1,1,1,1,4),(15.7079632679489,15.8838097603743,16.8712669125496,17.8587240647249,
18.8461812169001,19.8336383690754,20.8210955212507,21.808552673426,21.9911485751285),
 .UNSPECIFIED.);
#559=B_SPLINE_CURVE_WITH_KNOTS('',3,(#39108,#39109,#39110,#39111,#39112,
#39113,#39114,#39115,#39116,#39117),.UNSPECIFIED.,.F.,.F.,(4,1,1,1,1,1,
1,4),(15.7079632679489,16.5247731074507,17.512230259626,18.4996874118013,
19.4871445639766,20.4746017161519,21.4620588683272,21.9911485751285),
 .UNSPECIFIED.);
#560=B_SPLINE_CURVE_WITH_KNOTS('',3,(#39343,#39344,#39345,#39346,#39347,
#39348,#39349,#39350,#39351,#39352,#39353,#39354,#39355,#39356,#39357,#39358,
#39359,#39360,#39361,#39362,#39363,#39364,#39365,#39366,#39367,#39368,#39369,
#39370,#39371,#39372,#39373,#39374,#39375,#39376,#39377,#39378,#39379,#39380,
#39381,#39382,#39383,#39384,#39385,#39386,#39387,#39388,#39389,#39390,#39391),
 .UNSPECIFIED.,.F.,.F.,(4,3,3,3,3,3,3,3,3,3,3,3,3,3,3,3,4),(-0.226379821609611,
-0.214890180424997,-0.195063355378614,-0.183728168968286,-0.169237877031892,
-0.156768292348793,-0.131336338642949,-0.121264777035684,-0.11376486268334,
-0.101603376860372,-0.0859957740860565,-0.07722199741945,-0.0531920110136073,
-0.041845954216628,-0.0323163699760562,-0.00989131159632156,0.),
 .UNSPECIFIED.);
#561=B_SPLINE_CURVE_WITH_KNOTS('',3,(#39392,#39393,#39394,#39395,#39396,
#39397,#39398,#39399,#39400,#39401),.UNSPECIFIED.,.F.,.F.,(4,3,3,4),(48.1027730716318,
48.3854004565894,49.3728576087647,50.2654824574367),.UNSPECIFIED.);
#562=B_SPLINE_CURVE_WITH_KNOTS('',3,(#39403,#39404,#39405,#39406,#39407,
#39408,#39409,#39410,#39411,#39412,#39413,#39414,#39415,#39416,#39417,#39418,
#39419,#39420,#39421,#39422,#39423,#39424,#39425,#39426,#39427,#39428,#39429,
#39430,#39431,#39432,#39433,#39434,#39435,#39436,#39437,#39438,#39439,#39440,
#39441,#39442,#39443,#39444,#39445,#39446,#39447,#39448,#39449,#39450,#39451),
 .UNSPECIFIED.,.F.,.F.,(4,3,3,3,3,3,3,3,3,3,3,3,3,3,3,3,4),(-0.227523845437318,
-0.218254285946759,-0.205376019353374,-0.194839584423376,-0.181726252813619,
-0.172870003901879,-0.148477559368614,-0.136842916469509,-0.12791553259114,
-0.115084966565271,-0.0973336680873777,-0.0847825202648984,-0.0635868901986738,
-0.0502811887773191,-0.0410407821760877,-0.014115200632659,0.),
 .UNSPECIFIED.);
#563=B_SPLINE_CURVE_WITH_KNOTS('',3,(#39452,#39453,#39454,#39455,#39456,
#39457),.UNSPECIFIED.,.F.,.F.,(4,1,1,4),(13.6572339544282,14.5498588031001,
15.5373159552754,15.7079632679489),.UNSPECIFIED.);
#564=B_SPLINE_CURVE_WITH_KNOTS('',3,(#39460,#39461,#39462,#39463,#39464,
#39465,#39466,#39467,#39468,#39469,#39470,#39471,#39472,#39473,#39474,#39475,
#39476,#39477,#39478,#39479,#39480,#39481,#39482,#39483,#39484,#39485,#39486,
#39487,#39488,#39489,#39490,#39491,#39492,#39493,#39494,#39495,#39496,#39497,
#39498,#39499,#39500,#39501,#39502,#39503,#39504,#39505,#39506,#39507,#39508),
 .UNSPECIFIED.,.F.,.F.,(4,3,3,3,3,3,3,3,3,3,3,3,3,3,3,3,4),(-0.226379821609596,
-0.214890180424979,-0.195063350039947,-0.183728164322639,-0.169237850825561,
-0.156768290223532,-0.131336328824517,-0.12126472687929,-0.113764786721133,
-0.101603376860369,-0.0859957671104269,-0.0772219948002901,-0.0531920146182027,
-0.0418459669675516,-0.0323163753079122,-0.00989133560397837,0.),
 .UNSPECIFIED.);
#565=B_SPLINE_CURVE_WITH_KNOTS('',3,(#39511,#39512,#39513,#39514),
 .UNSPECIFIED.,.F.,.F.,(4,4),(14.896352608199,15.7079632679489),
 .UNSPECIFIED.);
#566=B_SPLINE_CURVE_WITH_KNOTS('',3,(#39740,#39741,#39742,#39743,#39744,
#39745,#39746,#39747,#39748,#39749,#39750,#39751,#39752,#39753,#39754,#39755,
#39756,#39757,#39758,#39759,#39760,#39761,#39762,#39763,#39764,#39765,#39766,
#39767,#39768,#39769,#39770,#39771,#39772,#39773,#39774,#39775,#39776,#39777,
#39778,#39779,#39780,#39781,#39782,#39783,#39784,#39785,#39786,#39787,#39788),
 .UNSPECIFIED.,.F.,.F.,(4,3,3,3,3,3,3,3,3,3,3,3,3,3,3,3,4),(-0.227523845437314,
-0.218254285946756,-0.205376031384273,-0.194839581377744,-0.181726328485879,
-0.172870086995034,-0.148477642599549,-0.13684302479023,-0.127915530672829,
-0.11508496656527,-0.0973336777498854,-0.0847825188673741,-0.0635868891505306,
-0.050281187305254,-0.0410407836210242,-0.0141152073468077,0.),
 .UNSPECIFIED.);
#567=B_SPLINE_CURVE_WITH_KNOTS('',3,(#39789,#39790,#39791,#39792,#39793,
#39794,#39795),.UNSPECIFIED.,.F.,.F.,(4,3,4),(-52.3352290652906,-51.3477719131153,
-51.0770931171867),.UNSPECIFIED.);
#970=SHAPE_REPRESENTATION_RELATIONSHIP('SRR','None',#55118,#990);
#990=ADVANCED_BREP_SHAPE_REPRESENTATION('',(#1030),#54996);
#1010=STYLED_ITEM('',(#55379),#1030);
#1030=MANIFOLD_SOLID_BREP('Hex Standoff',#24543);
#1261=FACE_BOUND('',#4742,.T.);
#1262=FACE_BOUND('',#4755,.T.);
#1548=PLANE('',#26206);
#1549=PLANE('',#26229);
#1550=PLANE('',#26230);
#1551=PLANE('',#26231);
#1552=PLANE('',#26232);
#1553=PLANE('',#26233);
#1554=PLANE('',#26246);
#1555=PLANE('',#26247);
#1556=PLANE('',#26250);
#1557=PLANE('',#26251);
#2202=CYLINDRICAL_SURFACE('',#26186,0.1215);
#2203=CYLINDRICAL_SURFACE('',#26190,0.1215);
#2204=CYLINDRICAL_SURFACE('',#26191,0.1215);
#2205=CYLINDRICAL_SURFACE('',#26192,0.1215);
#2206=CYLINDRICAL_SURFACE('',#26193,0.1215);
#2207=CYLINDRICAL_SURFACE('',#26194,0.1215);
#2208=CYLINDRICAL_SURFACE('',#26195,0.1215);
#2209=CYLINDRICAL_SURFACE('',#26196,0.1215);
#2210=CYLINDRICAL_SURFACE('',#26197,0.095825);
#2211=CYLINDRICAL_SURFACE('',#26199,0.095825);
#2212=CYLINDRICAL_SURFACE('',#26200,0.095825);
#2213=CYLINDRICAL_SURFACE('',#26201,0.095825);
#2214=CYLINDRICAL_SURFACE('',#26202,0.095825);
#2215=CYLINDRICAL_SURFACE('',#26203,0.095825);
#2216=CYLINDRICAL_SURFACE('',#26204,0.095825);
#2217=CYLINDRICAL_SURFACE('',#26205,0.095825);
#2218=CYLINDRICAL_SURFACE('',#26208,0.095825);
#2219=CYLINDRICAL_SURFACE('',#26209,0.1215);
#2220=CYLINDRICAL_SURFACE('',#26213,0.13);
#3119=FACE_OUTER_BOUND('',#4708,.T.);
#3120=FACE_OUTER_BOUND('',#4709,.T.);
#3121=FACE_OUTER_BOUND('',#4710,.T.);
#3122=FACE_OUTER_BOUND('',#4711,.T.);
#3123=FACE_OUTER_BOUND('',#4712,.T.);
#3124=FACE_OUTER_BOUND('',#4713,.T.);
#3125=FACE_OUTER_BOUND('',#4714,.T.);
#3126=FACE_OUTER_BOUND('',#4715,.T.);
#3127=FACE_OUTER_BOUND('',#4716,.T.);
#3128=FACE_OUTER_BOUND('',#4717,.T.);
#3129=FACE_OUTER_BOUND('',#4718,.T.);
#3130=FACE_OUTER_BOUND('',#4719,.T.);
#3131=FACE_OUTER_BOUND('',#4720,.T.);
#3132=FACE_OUTER_BOUND('',#4721,.T.);
#3133=FACE_OUTER_BOUND('',#4722,.T.);
#3134=FACE_OUTER_BOUND('',#4723,.T.);
#3135=FACE_OUTER_BOUND('',#4724,.T.);
#3136=FACE_OUTER_BOUND('',#4725,.T.);
#3137=FACE_OUTER_BOUND('',#4726,.T.);
#3138=FACE_OUTER_BOUND('',#4727,.T.);
#3139=FACE_OUTER_BOUND('',#4728,.T.);
#3140=FACE_OUTER_BOUND('',#4729,.T.);
#3141=FACE_OUTER_BOUND('',#4730,.T.);
#3142=FACE_OUTER_BOUND('',#4731,.T.);
#3143=FACE_OUTER_BOUND('',#4732,.T.);
#3144=FACE_OUTER_BOUND('',#4733,.T.);
#3145=FACE_OUTER_BOUND('',#4734,.T.);
#3146=FACE_OUTER_BOUND('',#4735,.T.);
#3147=FACE_OUTER_BOUND('',#4736,.T.);
#3148=FACE_OUTER_BOUND('',#4737,.T.);
#3149=FACE_OUTER_BOUND('',#4738,.T.);
#3150=FACE_OUTER_BOUND('',#4739,.T.);
#3151=FACE_OUTER_BOUND('',#4740,.T.);
#3152=FACE_OUTER_BOUND('',#4741,.T.);
#3153=FACE_OUTER_BOUND('',#4743,.T.);
#3154=FACE_OUTER_BOUND('',#4744,.T.);
#3155=FACE_OUTER_BOUND('',#4745,.T.);
#3156=FACE_OUTER_BOUND('',#4746,.T.);
#3157=FACE_OUTER_BOUND('',#4747,.T.);
#3158=FACE_OUTER_BOUND('',#4748,.T.);
#3159=FACE_OUTER_BOUND('',#4749,.T.);
#3160=FACE_OUTER_BOUND('',#4750,.T.);
#3161=FACE_OUTER_BOUND('',#4751,.T.);
#3162=FACE_OUTER_BOUND('',#4752,.T.);
#3163=FACE_OUTER_BOUND('',#4753,.T.);
#3164=FACE_OUTER_BOUND('',#4754,.T.);
#4708=EDGE_LOOP('',(#19198,#19199,#19200,#19201,#19202,#19203,#19204,#19205));
#4709=EDGE_LOOP('',(#19206,#19207,#19208,#19209));
#4710=EDGE_LOOP('',(#19210,#19211,#19212,#19213));
#4711=EDGE_LOOP('',(#19214,#19215,#19216,#19217));
#4712=EDGE_LOOP('',(#19218,#19219,#19220,#19221));
#4713=EDGE_LOOP('',(#19222,#19223,#19224,#19225));
#4714=EDGE_LOOP('',(#19226,#19227,#19228,#19229));
#4715=EDGE_LOOP('',(#19230,#19231,#19232,#19233));
#4716=EDGE_LOOP('',(#19234,#19235,#19236,#19237));
#4717=EDGE_LOOP('',(#19238,#19239,#19240,#19241));
#4718=EDGE_LOOP('',(#19242,#19243,#19244,#19245));
#4719=EDGE_LOOP('',(#19246,#19247,#19248,#19249));
#4720=EDGE_LOOP('',(#19250,#19251,#19252,#19253));
#4721=EDGE_LOOP('',(#19254,#19255,#19256,#19257));
#4722=EDGE_LOOP('',(#19258,#19259,#19260,#19261));
#4723=EDGE_LOOP('',(#19262,#19263,#19264,#19265));
#4724=EDGE_LOOP('',(#19266,#19267,#19268,#19269,#19270,#19271,#19272,#19273,
#19274,#19275,#19276,#19277,#19278,#19279,#19280,#19281,#19282,#19283,#19284,
#19285));
#4725=EDGE_LOOP('',(#19286,#19287,#19288,#19289,#19290));
#4726=EDGE_LOOP('',(#19291,#19292,#19293,#19294));
#4727=EDGE_LOOP('',(#19295,#19296,#19297,#19298,#19299,#19300,#19301,#19302,
#19303,#19304,#19305,#19306,#19307,#19308,#19309,#19310,#19311,#19312,#19313,
#19314));
#4728=EDGE_LOOP('',(#19315,#19316,#19317,#19318));
#4729=EDGE_LOOP('',(#19319,#19320,#19321));
#4730=EDGE_LOOP('',(#19322,#19323,#19324,#19325));
#4731=EDGE_LOOP('',(#19326,#19327,#19328,#19329));
#4732=EDGE_LOOP('',(#19330,#19331,#19332));
#4733=EDGE_LOOP('',(#19333,#19334,#19335));
#4734=EDGE_LOOP('',(#19336,#19337,#19338));
#4735=EDGE_LOOP('',(#19339,#19340,#19341));
#4736=EDGE_LOOP('',(#19342,#19343,#19344));
#4737=EDGE_LOOP('',(#19345,#19346,#19347));
#4738=EDGE_LOOP('',(#19348,#19349,#19350,#19351,#19352,#19353,#19354,#19355));
#4739=EDGE_LOOP('',(#19356,#19357,#19358,#19359,#19360,#19361,#19362,#19363));
#4740=EDGE_LOOP('',(#19364,#19365,#19366,#19367,#19368,#19369,#19370,#19371));
#4741=EDGE_LOOP('',(#19372,#19373,#19374,#19375,#19376,#19377,#19378,#19379,
#19380,#19381,#19382,#19383));
#4742=EDGE_LOOP('',(#19384,#19385,#19386,#19387));
#4743=EDGE_LOOP('',(#19388,#19389,#19390,#19391,#19392,#19393,#19394,#19395));
#4744=EDGE_LOOP('',(#19396,#19397,#19398));
#4745=EDGE_LOOP('',(#19399,#19400,#19401));
#4746=EDGE_LOOP('',(#19402,#19403,#19404));
#4747=EDGE_LOOP('',(#19405,#19406,#19407));
#4748=EDGE_LOOP('',(#19408,#19409,#19410));
#4749=EDGE_LOOP('',(#19411,#19412,#19413));
#4750=EDGE_LOOP('',(#19414,#19415,#19416,#19417,#19418,#19419,#19420,#19421));
#4751=EDGE_LOOP('',(#19422));
#4752=EDGE_LOOP('',(#19423,#19424,#19425,#19426));
#4753=EDGE_LOOP('',(#19427,#19428,#19429,#19430,#19431,#19432,#19433,#19434));
#4754=EDGE_LOOP('',(#19435,#19436,#19437,#19438,#19439,#19440,#19441,#19442,
#19443,#19444,#19445,#19446));
#4755=EDGE_LOOP('',(#19447));
#6294=LINE('',#38532,#8115);
#6295=LINE('',#38556,#8116);
#6296=LINE('',#38579,#8117);
#6297=LINE('',#38627,#8118);
#6298=LINE('',#38675,#8119);
#6299=LINE('',#38729,#8120);
#6300=LINE('',#38777,#8121);
#6301=LINE('',#38825,#8122);
#6302=LINE('',#38876,#8123);
#6303=LINE('',#38924,#8124);
#6304=LINE('',#38948,#8125);
#6305=LINE('',#38973,#8126);
#6306=LINE('',#38998,#8127);
#6307=LINE('',#39022,#8128);
#6308=LINE('',#39047,#8129);
#6309=LINE('',#39072,#8130);
#6310=LINE('',#39096,#8131);
#6311=LINE('',#39801,#8132);
#6312=LINE('',#39805,#8133);
#6313=LINE('',#39809,#8134);
#6314=LINE('',#39879,#8135);
#6315=LINE('',#39885,#8136);
#6316=LINE('',#39890,#8137);
#6317=LINE('',#39891,#8138);
#6318=LINE('',#39898,#8139);
#6319=LINE('',#39903,#8140);
#6320=LINE('',#39904,#8141);
#6321=LINE('',#39911,#8142);
#6322=LINE('',#39916,#8143);
#6323=LINE('',#39917,#8144);
#6324=LINE('',#39919,#8145);
#6325=LINE('',#39920,#8146);
#6326=LINE('',#39921,#8147);
#6327=LINE('',#39928,#8148);
#6328=LINE('',#39933,#8149);
#6329=LINE('',#39964,#8150);
#6330=LINE('',#39965,#8151);
#6331=LINE('',#39970,#8152);
#6332=LINE('',#39972,#8153);
#8115=VECTOR('',#30944,0.125);
#8116=VECTOR('',#30947,0.125);
#8117=VECTOR('',#30954,0.125);
#8118=VECTOR('',#30957,0.125);
#8119=VECTOR('',#30960,0.125);
#8120=VECTOR('',#30963,0.125);
#8121=VECTOR('',#30966,0.125);
#8122=VECTOR('',#30969,0.125);
#8123=VECTOR('',#30972,0.125);
#8124=VECTOR('',#30975,0.095825);
#8125=VECTOR('',#30980,0.095825);
#8126=VECTOR('',#30983,0.095825);
#8127=VECTOR('',#30986,0.095825);
#8128=VECTOR('',#30989,0.095825);
#8129=VECTOR('',#30992,0.095825);
#8130=VECTOR('',#30995,0.095825);
#8131=VECTOR('',#30998,0.095825);
#8132=VECTOR('',#31011,0.065);
#8133=VECTOR('',#31016,0.13);
#8134=VECTOR('',#31021,0.18);
#8135=VECTOR('',#31050,1.);
#8136=VECTOR('',#31051,1.);
#8137=VECTOR('',#31052,1.);
#8138=VECTOR('',#31053,1.);
#8139=VECTOR('',#31056,1.);
#8140=VECTOR('',#31057,1.);
#8141=VECTOR('',#31058,1.);
#8142=VECTOR('',#31061,1.);
#8143=VECTOR('',#31062,1.);
#8144=VECTOR('',#31063,1.);
#8145=VECTOR('',#31066,1.);
#8146=VECTOR('',#31067,1.);
#8147=VECTOR('',#31068,1.);
#8148=VECTOR('',#31071,1.);
#8149=VECTOR('',#31072,1.);
#8150=VECTOR('',#31099,1.);
#8151=VECTOR('',#31100,1.);
#8152=VECTOR('',#31107,0.115);
#8153=VECTOR('',#31110,1.);
#9720=CIRCLE('',#26187,0.1215);
#9721=CIRCLE('',#26188,0.1215);
#9722=CIRCLE('',#26189,0.1215);
#9723=CIRCLE('',#26198,0.095825);
#9724=CIRCLE('',#26207,0.095825);
#9725=CIRCLE('',#26210,0.1215);
#9726=CIRCLE('',#26212,0.13);
#9727=CIRCLE('',#26214,0.13);
#9728=CIRCLE('',#26216,0.18);
#9729=CIRCLE('',#26218,0.255);
#9730=CIRCLE('',#26220,0.255);
#9731=CIRCLE('',#26222,0.255);
#9732=CIRCLE('',#26224,0.255);
#9733=CIRCLE('',#26226,0.255);
#9734=CIRCLE('',#26228,0.255);
#9735=CIRCLE('',#26235,0.255);
#9736=CIRCLE('',#26237,0.255);
#9737=CIRCLE('',#26239,0.255);
#9738=CIRCLE('',#26241,0.255);
#9739=CIRCLE('',#26243,0.255);
#9740=CIRCLE('',#26245,0.255);
#9741=CIRCLE('',#26248,0.105);
#11102=VERTEX_POINT('',#38530);
#11103=VERTEX_POINT('',#38531);
#11104=VERTEX_POINT('',#38533);
#11105=VERTEX_POINT('',#38553);
#11106=VERTEX_POINT('',#38555);
#11107=VERTEX_POINT('',#38558);
#11108=VERTEX_POINT('',#38577);
#11109=VERTEX_POINT('',#38578);
#11110=VERTEX_POINT('',#38625);
#11111=VERTEX_POINT('',#38626);
#11112=VERTEX_POINT('',#38673);
#11113=VERTEX_POINT('',#38674);
#11114=VERTEX_POINT('',#38727);
#11115=VERTEX_POINT('',#38728);
#11116=VERTEX_POINT('',#38775);
#11117=VERTEX_POINT('',#38776);
#11118=VERTEX_POINT('',#38823);
#11119=VERTEX_POINT('',#38824);
#11120=VERTEX_POINT('',#38874);
#11121=VERTEX_POINT('',#38875);
#11122=VERTEX_POINT('',#38922);
#11123=VERTEX_POINT('',#38923);
#11124=VERTEX_POINT('',#38925);
#11125=VERTEX_POINT('',#38935);
#11126=VERTEX_POINT('',#38946);
#11127=VERTEX_POINT('',#38947);
#11128=VERTEX_POINT('',#38971);
#11129=VERTEX_POINT('',#38972);
#11130=VERTEX_POINT('',#38996);
#11131=VERTEX_POINT('',#38997);
#11132=VERTEX_POINT('',#39020);
#11133=VERTEX_POINT('',#39021);
#11134=VERTEX_POINT('',#39045);
#11135=VERTEX_POINT('',#39046);
#11136=VERTEX_POINT('',#39070);
#11137=VERTEX_POINT('',#39071);
#11138=VERTEX_POINT('',#39094);
#11139=VERTEX_POINT('',#39095);
#11140=VERTEX_POINT('',#39342);
#11141=VERTEX_POINT('',#39402);
#11142=VERTEX_POINT('',#39459);
#11143=VERTEX_POINT('',#39739);
#11144=VERTEX_POINT('',#39799);
#11145=VERTEX_POINT('',#39800);
#11146=VERTEX_POINT('',#39804);
#11147=VERTEX_POINT('',#39808);
#11148=VERTEX_POINT('',#39812);
#11149=VERTEX_POINT('',#39813);
#11150=VERTEX_POINT('',#39817);
#11151=VERTEX_POINT('',#39823);
#11152=VERTEX_POINT('',#39824);
#11153=VERTEX_POINT('',#39828);
#11154=VERTEX_POINT('',#39834);
#11155=VERTEX_POINT('',#39835);
#11156=VERTEX_POINT('',#39839);
#11157=VERTEX_POINT('',#39845);
#11158=VERTEX_POINT('',#39846);
#11159=VERTEX_POINT('',#39850);
#11160=VERTEX_POINT('',#39856);
#11161=VERTEX_POINT('',#39857);
#11162=VERTEX_POINT('',#39861);
#11163=VERTEX_POINT('',#39867);
#11164=VERTEX_POINT('',#39868);
#11165=VERTEX_POINT('',#39872);
#11166=VERTEX_POINT('',#39878);
#11167=VERTEX_POINT('',#39880);
#11168=VERTEX_POINT('',#39884);
#11169=VERTEX_POINT('',#39886);
#11170=VERTEX_POINT('',#39893);
#11171=VERTEX_POINT('',#39897);
#11172=VERTEX_POINT('',#39899);
#11173=VERTEX_POINT('',#39906);
#11174=VERTEX_POINT('',#39910);
#11175=VERTEX_POINT('',#39912);
#11176=VERTEX_POINT('',#39923);
#11177=VERTEX_POINT('',#39927);
#11178=VERTEX_POINT('',#39929);
#11179=VERTEX_POINT('',#39935);
#11180=VERTEX_POINT('',#39936);
#11181=VERTEX_POINT('',#39940);
#11182=VERTEX_POINT('',#39946);
#11183=VERTEX_POINT('',#39958);
#11184=VERTEX_POINT('',#39967);
#14007=EDGE_CURVE('',#11102,#11103,#6294,.T.);
#14008=EDGE_CURVE('',#11102,#11104,#528,.T.);
#14009=EDGE_CURVE('',#11104,#11105,#9720,.T.);
#14010=EDGE_CURVE('',#11105,#11106,#6295,.T.);
#14011=EDGE_CURVE('',#11106,#11106,#9721,.T.);
#14012=EDGE_CURVE('',#11105,#11107,#9722,.T.);
#14013=EDGE_CURVE('',#11107,#11103,#529,.T.);
#14014=EDGE_CURVE('',#11108,#11109,#6296,.T.);
#14015=EDGE_CURVE('',#11108,#11102,#530,.T.);
#14016=EDGE_CURVE('',#11103,#11109,#531,.T.);
#14017=EDGE_CURVE('',#11110,#11111,#6297,.T.);
#14018=EDGE_CURVE('',#11110,#11108,#532,.T.);
#14019=EDGE_CURVE('',#11109,#11111,#533,.T.);
#14020=EDGE_CURVE('',#11112,#11113,#6298,.T.);
#14021=EDGE_CURVE('',#11112,#11110,#534,.T.);
#14022=EDGE_CURVE('',#11111,#11113,#535,.T.);
#14023=EDGE_CURVE('',#11114,#11115,#6299,.T.);
#14024=EDGE_CURVE('',#11114,#11112,#536,.T.);
#14025=EDGE_CURVE('',#11113,#11115,#537,.T.);
#14026=EDGE_CURVE('',#11116,#11117,#6300,.T.);
#14027=EDGE_CURVE('',#11116,#11114,#538,.T.);
#14028=EDGE_CURVE('',#11115,#11117,#539,.T.);
#14029=EDGE_CURVE('',#11118,#11119,#6301,.T.);
#14030=EDGE_CURVE('',#11118,#11116,#540,.T.);
#14031=EDGE_CURVE('',#11117,#11119,#541,.T.);
#14032=EDGE_CURVE('',#11120,#11121,#6302,.T.);
#14033=EDGE_CURVE('',#11120,#11118,#542,.T.);
#14034=EDGE_CURVE('',#11119,#11121,#543,.T.);
#14035=EDGE_CURVE('',#11122,#11123,#6303,.T.);
#14036=EDGE_CURVE('',#11122,#11124,#544,.T.);
#14037=EDGE_CURVE('',#11125,#11124,#9723,.T.);
#14038=EDGE_CURVE('',#11123,#11125,#545,.T.);
#14039=EDGE_CURVE('',#11126,#11127,#6304,.T.);
#14040=EDGE_CURVE('',#11126,#11122,#546,.T.);
#14041=EDGE_CURVE('',#11127,#11123,#547,.T.);
#14042=EDGE_CURVE('',#11128,#11129,#6305,.T.);
#14043=EDGE_CURVE('',#11128,#11126,#548,.T.);
#14044=EDGE_CURVE('',#11129,#11127,#549,.T.);
#14045=EDGE_CURVE('',#11130,#11131,#6306,.T.);
#14046=EDGE_CURVE('',#11130,#11128,#550,.T.);
#14047=EDGE_CURVE('',#11131,#11129,#551,.T.);
#14048=EDGE_CURVE('',#11132,#11133,#6307,.T.);
#14049=EDGE_CURVE('',#11132,#11130,#552,.T.);
#14050=EDGE_CURVE('',#11133,#11131,#553,.T.);
#14051=EDGE_CURVE('',#11134,#11135,#6308,.T.);
#14052=EDGE_CURVE('',#11134,#11132,#554,.T.);
#14053=EDGE_CURVE('',#11135,#11133,#555,.T.);
#14054=EDGE_CURVE('',#11136,#11137,#6309,.T.);
#14055=EDGE_CURVE('',#11136,#11134,#556,.T.);
#14056=EDGE_CURVE('',#11137,#11135,#557,.T.);
#14057=EDGE_CURVE('',#11138,#11139,#6310,.T.);
#14058=EDGE_CURVE('',#11138,#11136,#558,.T.);
#14059=EDGE_CURVE('',#11139,#11137,#559,.T.);
#14060=EDGE_CURVE('',#11140,#11125,#560,.T.);
#14061=EDGE_CURVE('',#11121,#11140,#561,.T.);
#14062=EDGE_CURVE('',#11141,#11107,#562,.T.);
#14063=EDGE_CURVE('',#11141,#11139,#563,.T.);
#14064=EDGE_CURVE('',#11104,#11142,#564,.T.);
#14065=EDGE_CURVE('',#11142,#11141,#9724,.T.);
#14066=EDGE_CURVE('',#11142,#11138,#565,.T.);
#14067=EDGE_CURVE('',#11124,#11143,#566,.T.);
#14068=EDGE_CURVE('',#11143,#11120,#567,.T.);
#14069=EDGE_CURVE('',#11143,#11140,#9725,.F.);
#14070=EDGE_CURVE('',#11144,#11145,#6311,.T.);
#14071=EDGE_CURVE('',#11145,#11145,#9726,.T.);
#14072=EDGE_CURVE('',#11145,#11146,#6312,.T.);
#14073=EDGE_CURVE('',#11146,#11146,#9727,.T.);
#14074=EDGE_CURVE('',#11146,#11147,#6313,.T.);
#14075=EDGE_CURVE('',#11147,#11147,#9728,.T.);
#14076=EDGE_CURVE('',#11148,#11149,#227,.T.);
#14077=EDGE_CURVE('',#11150,#11148,#228,.T.);
#14078=EDGE_CURVE('',#11149,#11150,#9729,.T.);
#14079=EDGE_CURVE('',#11151,#11152,#229,.T.);
#14080=EDGE_CURVE('',#11153,#11151,#230,.T.);
#14081=EDGE_CURVE('',#11152,#11153,#9730,.T.);
#14082=EDGE_CURVE('',#11154,#11155,#231,.T.);
#14083=EDGE_CURVE('',#11156,#11154,#232,.T.);
#14084=EDGE_CURVE('',#11155,#11156,#9731,.T.);
#14085=EDGE_CURVE('',#11157,#11158,#233,.T.);
#14086=EDGE_CURVE('',#11159,#11157,#234,.T.);
#14087=EDGE_CURVE('',#11158,#11159,#9732,.T.);
#14088=EDGE_CURVE('',#11160,#11161,#235,.T.);
#14089=EDGE_CURVE('',#11162,#11160,#236,.T.);
#14090=EDGE_CURVE('',#11161,#11162,#9733,.T.);
#14091=EDGE_CURVE('',#11163,#11164,#237,.T.);
#14092=EDGE_CURVE('',#11165,#11163,#9734,.T.);
#14093=EDGE_CURVE('',#11164,#11165,#238,.T.);
#14094=EDGE_CURVE('',#11160,#11166,#6314,.T.);
#14095=EDGE_CURVE('',#11166,#11167,#239,.T.);
#14096=EDGE_CURVE('',#11168,#11167,#6315,.T.);
#14097=EDGE_CURVE('',#11168,#11169,#240,.T.);
#14098=EDGE_CURVE('',#11157,#11169,#6316,.T.);
#14099=EDGE_CURVE('',#11158,#11162,#6317,.T.);
#14100=EDGE_CURVE('',#11169,#11170,#241,.T.);
#14101=EDGE_CURVE('',#11171,#11170,#6318,.T.);
#14102=EDGE_CURVE('',#11171,#11172,#242,.T.);
#14103=EDGE_CURVE('',#11154,#11172,#6319,.T.);
#14104=EDGE_CURVE('',#11155,#11159,#6320,.T.);
#14105=EDGE_CURVE('',#11172,#11173,#243,.T.);
#14106=EDGE_CURVE('',#11174,#11173,#6321,.T.);
#14107=EDGE_CURVE('',#11174,#11175,#244,.T.);
#14108=EDGE_CURVE('',#11151,#11175,#6322,.T.);
#14109=EDGE_CURVE('',#11152,#11156,#6323,.T.);
#14110=EDGE_CURVE('',#11161,#11163,#6324,.T.);
#14111=EDGE_CURVE('',#11149,#11153,#6325,.T.);
#14112=EDGE_CURVE('',#11165,#11150,#6326,.T.);
#14113=EDGE_CURVE('',#11175,#11176,#245,.T.);
#14114=EDGE_CURVE('',#11177,#11176,#6327,.T.);
#14115=EDGE_CURVE('',#11177,#11178,#246,.T.);
#14116=EDGE_CURVE('',#11148,#11178,#6328,.T.);
#14117=EDGE_CURVE('',#11179,#11180,#247,.T.);
#14118=EDGE_CURVE('',#11181,#11179,#9735,.T.);
#14119=EDGE_CURVE('',#11180,#11181,#248,.T.);
#14120=EDGE_CURVE('',#11182,#11177,#9736,.T.);
#14121=EDGE_CURVE('',#11178,#11182,#249,.T.);
#14122=EDGE_CURVE('',#11176,#11174,#9737,.T.);
#14123=EDGE_CURVE('',#11173,#11171,#9738,.T.);
#14124=EDGE_CURVE('',#11170,#11168,#9739,.T.);
#14125=EDGE_CURVE('',#11183,#11166,#250,.T.);
#14126=EDGE_CURVE('',#11167,#11183,#9740,.T.);
#14127=EDGE_CURVE('',#11164,#11180,#6329,.T.);
#14128=EDGE_CURVE('',#11183,#11181,#6330,.T.);
#14129=EDGE_CURVE('',#11184,#11184,#9741,.T.);
#14130=EDGE_CURVE('',#11106,#11184,#6331,.T.);
#14131=EDGE_CURVE('',#11179,#11182,#6332,.T.);
#19198=ORIENTED_EDGE('',*,*,#14007,.F.);
#19199=ORIENTED_EDGE('',*,*,#14008,.T.);
#19200=ORIENTED_EDGE('',*,*,#14009,.T.);
#19201=ORIENTED_EDGE('',*,*,#14010,.T.);
#19202=ORIENTED_EDGE('',*,*,#14011,.T.);
#19203=ORIENTED_EDGE('',*,*,#14010,.F.);
#19204=ORIENTED_EDGE('',*,*,#14012,.T.);
#19205=ORIENTED_EDGE('',*,*,#14013,.T.);
#19206=ORIENTED_EDGE('',*,*,#14014,.F.);
#19207=ORIENTED_EDGE('',*,*,#14015,.T.);
#19208=ORIENTED_EDGE('',*,*,#14007,.T.);
#19209=ORIENTED_EDGE('',*,*,#14016,.T.);
#19210=ORIENTED_EDGE('',*,*,#14017,.F.);
#19211=ORIENTED_EDGE('',*,*,#14018,.T.);
#19212=ORIENTED_EDGE('',*,*,#14014,.T.);
#19213=ORIENTED_EDGE('',*,*,#14019,.T.);
#19214=ORIENTED_EDGE('',*,*,#14020,.F.);
#19215=ORIENTED_EDGE('',*,*,#14021,.T.);
#19216=ORIENTED_EDGE('',*,*,#14017,.T.);
#19217=ORIENTED_EDGE('',*,*,#14022,.T.);
#19218=ORIENTED_EDGE('',*,*,#14023,.F.);
#19219=ORIENTED_EDGE('',*,*,#14024,.T.);
#19220=ORIENTED_EDGE('',*,*,#14020,.T.);
#19221=ORIENTED_EDGE('',*,*,#14025,.T.);
#19222=ORIENTED_EDGE('',*,*,#14026,.F.);
#19223=ORIENTED_EDGE('',*,*,#14027,.T.);
#19224=ORIENTED_EDGE('',*,*,#14023,.T.);
#19225=ORIENTED_EDGE('',*,*,#14028,.T.);
#19226=ORIENTED_EDGE('',*,*,#14029,.F.);
#19227=ORIENTED_EDGE('',*,*,#14030,.T.);
#19228=ORIENTED_EDGE('',*,*,#14026,.T.);
#19229=ORIENTED_EDGE('',*,*,#14031,.T.);
#19230=ORIENTED_EDGE('',*,*,#14032,.F.);
#19231=ORIENTED_EDGE('',*,*,#14033,.T.);
#19232=ORIENTED_EDGE('',*,*,#14029,.T.);
#19233=ORIENTED_EDGE('',*,*,#14034,.T.);
#19234=ORIENTED_EDGE('',*,*,#14035,.F.);
#19235=ORIENTED_EDGE('',*,*,#14036,.T.);
#19236=ORIENTED_EDGE('',*,*,#14037,.F.);
#19237=ORIENTED_EDGE('',*,*,#14038,.F.);
#19238=ORIENTED_EDGE('',*,*,#14039,.F.);
#19239=ORIENTED_EDGE('',*,*,#14040,.T.);
#19240=ORIENTED_EDGE('',*,*,#14035,.T.);
#19241=ORIENTED_EDGE('',*,*,#14041,.F.);
#19242=ORIENTED_EDGE('',*,*,#14042,.F.);
#19243=ORIENTED_EDGE('',*,*,#14043,.T.);
#19244=ORIENTED_EDGE('',*,*,#14039,.T.);
#19245=ORIENTED_EDGE('',*,*,#14044,.F.);
#19246=ORIENTED_EDGE('',*,*,#14045,.F.);
#19247=ORIENTED_EDGE('',*,*,#14046,.T.);
#19248=ORIENTED_EDGE('',*,*,#14042,.T.);
#19249=ORIENTED_EDGE('',*,*,#14047,.F.);
#19250=ORIENTED_EDGE('',*,*,#14048,.F.);
#19251=ORIENTED_EDGE('',*,*,#14049,.T.);
#19252=ORIENTED_EDGE('',*,*,#14045,.T.);
#19253=ORIENTED_EDGE('',*,*,#14050,.F.);
#19254=ORIENTED_EDGE('',*,*,#14051,.F.);
#19255=ORIENTED_EDGE('',*,*,#14052,.T.);
#19256=ORIENTED_EDGE('',*,*,#14048,.T.);
#19257=ORIENTED_EDGE('',*,*,#14053,.F.);
#19258=ORIENTED_EDGE('',*,*,#14054,.F.);
#19259=ORIENTED_EDGE('',*,*,#14055,.T.);
#19260=ORIENTED_EDGE('',*,*,#14051,.T.);
#19261=ORIENTED_EDGE('',*,*,#14056,.F.);
#19262=ORIENTED_EDGE('',*,*,#14057,.F.);
#19263=ORIENTED_EDGE('',*,*,#14058,.T.);
#19264=ORIENTED_EDGE('',*,*,#14054,.T.);
#19265=ORIENTED_EDGE('',*,*,#14059,.F.);
#19266=ORIENTED_EDGE('',*,*,#14060,.F.);
#19267=ORIENTED_EDGE('',*,*,#14061,.F.);
#19268=ORIENTED_EDGE('',*,*,#14034,.F.);
#19269=ORIENTED_EDGE('',*,*,#14031,.F.);
#19270=ORIENTED_EDGE('',*,*,#14028,.F.);
#19271=ORIENTED_EDGE('',*,*,#14025,.F.);
#19272=ORIENTED_EDGE('',*,*,#14022,.F.);
#19273=ORIENTED_EDGE('',*,*,#14019,.F.);
#19274=ORIENTED_EDGE('',*,*,#14016,.F.);
#19275=ORIENTED_EDGE('',*,*,#14013,.F.);
#19276=ORIENTED_EDGE('',*,*,#14062,.F.);
#19277=ORIENTED_EDGE('',*,*,#14063,.T.);
#19278=ORIENTED_EDGE('',*,*,#14059,.T.);
#19279=ORIENTED_EDGE('',*,*,#14056,.T.);
#19280=ORIENTED_EDGE('',*,*,#14053,.T.);
#19281=ORIENTED_EDGE('',*,*,#14050,.T.);
#19282=ORIENTED_EDGE('',*,*,#14047,.T.);
#19283=ORIENTED_EDGE('',*,*,#14044,.T.);
#19284=ORIENTED_EDGE('',*,*,#14041,.T.);
#19285=ORIENTED_EDGE('',*,*,#14038,.T.);
#19286=ORIENTED_EDGE('',*,*,#14009,.F.);
#19287=ORIENTED_EDGE('',*,*,#14064,.T.);
#19288=ORIENTED_EDGE('',*,*,#14065,.T.);
#19289=ORIENTED_EDGE('',*,*,#14062,.T.);
#19290=ORIENTED_EDGE('',*,*,#14012,.F.);
#19291=ORIENTED_EDGE('',*,*,#14057,.T.);
#19292=ORIENTED_EDGE('',*,*,#14063,.F.);
#19293=ORIENTED_EDGE('',*,*,#14065,.F.);
#19294=ORIENTED_EDGE('',*,*,#14066,.T.);
#19295=ORIENTED_EDGE('',*,*,#14067,.F.);
#19296=ORIENTED_EDGE('',*,*,#14036,.F.);
#19297=ORIENTED_EDGE('',*,*,#14040,.F.);
#19298=ORIENTED_EDGE('',*,*,#14043,.F.);
#19299=ORIENTED_EDGE('',*,*,#14046,.F.);
#19300=ORIENTED_EDGE('',*,*,#14049,.F.);
#19301=ORIENTED_EDGE('',*,*,#14052,.F.);
#19302=ORIENTED_EDGE('',*,*,#14055,.F.);
#19303=ORIENTED_EDGE('',*,*,#14058,.F.);
#19304=ORIENTED_EDGE('',*,*,#14066,.F.);
#19305=ORIENTED_EDGE('',*,*,#14064,.F.);
#19306=ORIENTED_EDGE('',*,*,#14008,.F.);
#19307=ORIENTED_EDGE('',*,*,#14015,.F.);
#19308=ORIENTED_EDGE('',*,*,#14018,.F.);
#19309=ORIENTED_EDGE('',*,*,#14021,.F.);
#19310=ORIENTED_EDGE('',*,*,#14024,.F.);
#19311=ORIENTED_EDGE('',*,*,#14027,.F.);
#19312=ORIENTED_EDGE('',*,*,#14030,.F.);
#19313=ORIENTED_EDGE('',*,*,#14033,.F.);
#19314=ORIENTED_EDGE('',*,*,#14068,.F.);
#19315=ORIENTED_EDGE('',*,*,#14032,.T.);
#19316=ORIENTED_EDGE('',*,*,#14061,.T.);
#19317=ORIENTED_EDGE('',*,*,#14069,.F.);
#19318=ORIENTED_EDGE('',*,*,#14068,.T.);
#19319=ORIENTED_EDGE('',*,*,#14070,.T.);
#19320=ORIENTED_EDGE('',*,*,#14071,.T.);
#19321=ORIENTED_EDGE('',*,*,#14070,.F.);
#19322=ORIENTED_EDGE('',*,*,#14071,.F.);
#19323=ORIENTED_EDGE('',*,*,#14072,.T.);
#19324=ORIENTED_EDGE('',*,*,#14073,.T.);
#19325=ORIENTED_EDGE('',*,*,#14072,.F.);
#19326=ORIENTED_EDGE('',*,*,#14073,.F.);
#19327=ORIENTED_EDGE('',*,*,#14074,.T.);
#19328=ORIENTED_EDGE('',*,*,#14075,.F.);
#19329=ORIENTED_EDGE('',*,*,#14074,.F.);
#19330=ORIENTED_EDGE('',*,*,#14076,.F.);
#19331=ORIENTED_EDGE('',*,*,#14077,.F.);
#19332=ORIENTED_EDGE('',*,*,#14078,.F.);
#19333=ORIENTED_EDGE('',*,*,#14079,.F.);
#19334=ORIENTED_EDGE('',*,*,#14080,.F.);
#19335=ORIENTED_EDGE('',*,*,#14081,.F.);
#19336=ORIENTED_EDGE('',*,*,#14082,.F.);
#19337=ORIENTED_EDGE('',*,*,#14083,.F.);
#19338=ORIENTED_EDGE('',*,*,#14084,.F.);
#19339=ORIENTED_EDGE('',*,*,#14085,.F.);
#19340=ORIENTED_EDGE('',*,*,#14086,.F.);
#19341=ORIENTED_EDGE('',*,*,#14087,.F.);
#19342=ORIENTED_EDGE('',*,*,#14088,.F.);
#19343=ORIENTED_EDGE('',*,*,#14089,.F.);
#19344=ORIENTED_EDGE('',*,*,#14090,.F.);
#19345=ORIENTED_EDGE('',*,*,#14091,.F.);
#19346=ORIENTED_EDGE('',*,*,#14092,.F.);
#19347=ORIENTED_EDGE('',*,*,#14093,.F.);
#19348=ORIENTED_EDGE('',*,*,#14089,.T.);
#19349=ORIENTED_EDGE('',*,*,#14094,.T.);
#19350=ORIENTED_EDGE('',*,*,#14095,.T.);
#19351=ORIENTED_EDGE('',*,*,#14096,.F.);
#19352=ORIENTED_EDGE('',*,*,#14097,.T.);
#19353=ORIENTED_EDGE('',*,*,#14098,.F.);
#19354=ORIENTED_EDGE('',*,*,#14085,.T.);
#19355=ORIENTED_EDGE('',*,*,#14099,.T.);
#19356=ORIENTED_EDGE('',*,*,#14086,.T.);
#19357=ORIENTED_EDGE('',*,*,#14098,.T.);
#19358=ORIENTED_EDGE('',*,*,#14100,.T.);
#19359=ORIENTED_EDGE('',*,*,#14101,.F.);
#19360=ORIENTED_EDGE('',*,*,#14102,.T.);
#19361=ORIENTED_EDGE('',*,*,#14103,.F.);
#19362=ORIENTED_EDGE('',*,*,#14082,.T.);
#19363=ORIENTED_EDGE('',*,*,#14104,.T.);
#19364=ORIENTED_EDGE('',*,*,#14083,.T.);
#19365=ORIENTED_EDGE('',*,*,#14103,.T.);
#19366=ORIENTED_EDGE('',*,*,#14105,.T.);
#19367=ORIENTED_EDGE('',*,*,#14106,.F.);
#19368=ORIENTED_EDGE('',*,*,#14107,.T.);
#19369=ORIENTED_EDGE('',*,*,#14108,.F.);
#19370=ORIENTED_EDGE('',*,*,#14079,.T.);
#19371=ORIENTED_EDGE('',*,*,#14109,.T.);
#19372=ORIENTED_EDGE('',*,*,#14092,.T.);
#19373=ORIENTED_EDGE('',*,*,#14110,.F.);
#19374=ORIENTED_EDGE('',*,*,#14090,.T.);
#19375=ORIENTED_EDGE('',*,*,#14099,.F.);
#19376=ORIENTED_EDGE('',*,*,#14087,.T.);
#19377=ORIENTED_EDGE('',*,*,#14104,.F.);
#19378=ORIENTED_EDGE('',*,*,#14084,.T.);
#19379=ORIENTED_EDGE('',*,*,#14109,.F.);
#19380=ORIENTED_EDGE('',*,*,#14081,.T.);
#19381=ORIENTED_EDGE('',*,*,#14111,.F.);
#19382=ORIENTED_EDGE('',*,*,#14078,.T.);
#19383=ORIENTED_EDGE('',*,*,#14112,.F.);
#19384=ORIENTED_EDGE('',*,*,#14069,.T.);
#19385=ORIENTED_EDGE('',*,*,#14060,.T.);
#19386=ORIENTED_EDGE('',*,*,#14037,.T.);
#19387=ORIENTED_EDGE('',*,*,#14067,.T.);
#19388=ORIENTED_EDGE('',*,*,#14080,.T.);
#19389=ORIENTED_EDGE('',*,*,#14108,.T.);
#19390=ORIENTED_EDGE('',*,*,#14113,.T.);
#19391=ORIENTED_EDGE('',*,*,#14114,.F.);
#19392=ORIENTED_EDGE('',*,*,#14115,.T.);
#19393=ORIENTED_EDGE('',*,*,#14116,.F.);
#19394=ORIENTED_EDGE('',*,*,#14076,.T.);
#19395=ORIENTED_EDGE('',*,*,#14111,.T.);
#19396=ORIENTED_EDGE('',*,*,#14117,.F.);
#19397=ORIENTED_EDGE('',*,*,#14118,.F.);
#19398=ORIENTED_EDGE('',*,*,#14119,.F.);
#19399=ORIENTED_EDGE('',*,*,#14115,.F.);
#19400=ORIENTED_EDGE('',*,*,#14120,.F.);
#19401=ORIENTED_EDGE('',*,*,#14121,.F.);
#19402=ORIENTED_EDGE('',*,*,#14107,.F.);
#19403=ORIENTED_EDGE('',*,*,#14122,.F.);
#19404=ORIENTED_EDGE('',*,*,#14113,.F.);
#19405=ORIENTED_EDGE('',*,*,#14102,.F.);
#19406=ORIENTED_EDGE('',*,*,#14123,.F.);
#19407=ORIENTED_EDGE('',*,*,#14105,.F.);
#19408=ORIENTED_EDGE('',*,*,#14097,.F.);
#19409=ORIENTED_EDGE('',*,*,#14124,.F.);
#19410=ORIENTED_EDGE('',*,*,#14100,.F.);
#19411=ORIENTED_EDGE('',*,*,#14095,.F.);
#19412=ORIENTED_EDGE('',*,*,#14125,.F.);
#19413=ORIENTED_EDGE('',*,*,#14126,.F.);
#19414=ORIENTED_EDGE('',*,*,#14091,.T.);
#19415=ORIENTED_EDGE('',*,*,#14127,.T.);
#19416=ORIENTED_EDGE('',*,*,#14119,.T.);
#19417=ORIENTED_EDGE('',*,*,#14128,.F.);
#19418=ORIENTED_EDGE('',*,*,#14125,.T.);
#19419=ORIENTED_EDGE('',*,*,#14094,.F.);
#19420=ORIENTED_EDGE('',*,*,#14088,.T.);
#19421=ORIENTED_EDGE('',*,*,#14110,.T.);
#19422=ORIENTED_EDGE('',*,*,#14129,.F.);
#19423=ORIENTED_EDGE('',*,*,#14011,.F.);
#19424=ORIENTED_EDGE('',*,*,#14130,.T.);
#19425=ORIENTED_EDGE('',*,*,#14129,.T.);
#19426=ORIENTED_EDGE('',*,*,#14130,.F.);
#19427=ORIENTED_EDGE('',*,*,#14093,.T.);
#19428=ORIENTED_EDGE('',*,*,#14112,.T.);
#19429=ORIENTED_EDGE('',*,*,#14077,.T.);
#19430=ORIENTED_EDGE('',*,*,#14116,.T.);
#19431=ORIENTED_EDGE('',*,*,#14121,.T.);
#19432=ORIENTED_EDGE('',*,*,#14131,.F.);
#19433=ORIENTED_EDGE('',*,*,#14117,.T.);
#19434=ORIENTED_EDGE('',*,*,#14127,.F.);
#19435=ORIENTED_EDGE('',*,*,#14126,.T.);
#19436=ORIENTED_EDGE('',*,*,#14128,.T.);
#19437=ORIENTED_EDGE('',*,*,#14118,.T.);
#19438=ORIENTED_EDGE('',*,*,#14131,.T.);
#19439=ORIENTED_EDGE('',*,*,#14120,.T.);
#19440=ORIENTED_EDGE('',*,*,#14114,.T.);
#19441=ORIENTED_EDGE('',*,*,#14122,.T.);
#19442=ORIENTED_EDGE('',*,*,#14106,.T.);
#19443=ORIENTED_EDGE('',*,*,#14123,.T.);
#19444=ORIENTED_EDGE('',*,*,#14101,.T.);
#19445=ORIENTED_EDGE('',*,*,#14124,.T.);
#19446=ORIENTED_EDGE('',*,*,#14096,.T.);
#19447=ORIENTED_EDGE('',*,*,#14075,.T.);
#23134=CONICAL_SURFACE('',#26211,0.065,1.02974425867665);
#23135=CONICAL_SURFACE('',#26215,0.18,0.785398163397448);
#23136=CONICAL_SURFACE('',#26217,0.2825,0.785398163397448);
#23137=CONICAL_SURFACE('',#26219,0.2825,0.785398163397448);
#23138=CONICAL_SURFACE('',#26221,0.2825,0.785398163397448);
#23139=CONICAL_SURFACE('',#26223,0.2825,0.785398163397448);
#23140=CONICAL_SURFACE('',#26225,0.2825,0.785398163397448);
#23141=CONICAL_SURFACE('',#26227,0.2825,0.785398163397448);
#23142=CONICAL_SURFACE('',#26234,0.2825,0.785398163397448);
#23143=CONICAL_SURFACE('',#26236,0.2825,0.785398163397448);
#23144=CONICAL_SURFACE('',#26238,0.2825,0.785398163397448);
#23145=CONICAL_SURFACE('',#26240,0.2825,0.785398163397448);
#23146=CONICAL_SURFACE('',#26242,0.2825,0.785398163397448);
#23147=CONICAL_SURFACE('',#26244,0.2825,0.785398163397448);
#23148=CONICAL_SURFACE('',#26249,0.115,0.785398163397448);
#23872=ADVANCED_FACE('',(#3119),#2202,.T.);
#23873=ADVANCED_FACE('',(#3120),#2203,.T.);
#23874=ADVANCED_FACE('',(#3121),#2204,.T.);
#23875=ADVANCED_FACE('',(#3122),#2205,.T.);
#23876=ADVANCED_FACE('',(#3123),#2206,.T.);
#23877=ADVANCED_FACE('',(#3124),#2207,.T.);
#23878=ADVANCED_FACE('',(#3125),#2208,.T.);
#23879=ADVANCED_FACE('',(#3126),#2209,.T.);
#23880=ADVANCED_FACE('',(#3127),#2210,.T.);
#23881=ADVANCED_FACE('',(#3128),#2211,.T.);
#23882=ADVANCED_FACE('',(#3129),#2212,.T.);
#23883=ADVANCED_FACE('',(#3130),#2213,.T.);
#23884=ADVANCED_FACE('',(#3131),#2214,.T.);
#23885=ADVANCED_FACE('',(#3132),#2215,.T.);
#23886=ADVANCED_FACE('',(#3133),#2216,.T.);
#23887=ADVANCED_FACE('',(#3134),#2217,.T.);
#23888=ADVANCED_FACE('',(#3135),#472,.F.);
#23889=ADVANCED_FACE('',(#3136),#1548,.T.);
#23890=ADVANCED_FACE('',(#3137),#2218,.T.);
#23891=ADVANCED_FACE('',(#3138),#473,.F.);
#23892=ADVANCED_FACE('',(#3139),#2219,.T.);
#23893=ADVANCED_FACE('',(#3140),#23134,.F.);
#23894=ADVANCED_FACE('',(#3141),#2220,.F.);
#23895=ADVANCED_FACE('',(#3142),#23135,.F.);
#23896=ADVANCED_FACE('',(#3143),#23136,.T.);
#23897=ADVANCED_FACE('',(#3144),#23137,.T.);
#23898=ADVANCED_FACE('',(#3145),#23138,.T.);
#23899=ADVANCED_FACE('',(#3146),#23139,.T.);
#23900=ADVANCED_FACE('',(#3147),#23140,.T.);
#23901=ADVANCED_FACE('',(#3148),#23141,.T.);
#23902=ADVANCED_FACE('',(#3149),#1549,.T.);
#23903=ADVANCED_FACE('',(#3150),#1550,.T.);
#23904=ADVANCED_FACE('',(#3151),#1551,.T.);
#23905=ADVANCED_FACE('',(#3152,#1261),#1552,.F.);
#23906=ADVANCED_FACE('',(#3153),#1553,.T.);
#23907=ADVANCED_FACE('',(#3154),#23142,.T.);
#23908=ADVANCED_FACE('',(#3155),#23143,.T.);
#23909=ADVANCED_FACE('',(#3156),#23144,.T.);
#23910=ADVANCED_FACE('',(#3157),#23145,.T.);
#23911=ADVANCED_FACE('',(#3158),#23146,.T.);
#23912=ADVANCED_FACE('',(#3159),#23147,.T.);
#23913=ADVANCED_FACE('',(#3160),#1554,.T.);
#23914=ADVANCED_FACE('',(#3161),#1555,.T.);
#23915=ADVANCED_FACE('',(#3162),#23148,.T.);
#23916=ADVANCED_FACE('',(#3163),#1556,.T.);
#23917=ADVANCED_FACE('',(#3164,#1262),#1557,.T.);
#24543=CLOSED_SHELL('',(#23872,#23873,#23874,#23875,#23876,#23877,#23878,
#23879,#23880,#23881,#23882,#23883,#23884,#23885,#23886,#23887,#23888,#23889,
#23890,#23891,#23892,#23893,#23894,#23895,#23896,#23897,#23898,#23899,#23900,
#23901,#23902,#23903,#23904,#23905,#23906,#23907,#23908,#23909,#23910,#23911,
#23912,#23913,#23914,#23915,#23916,#23917));
#26185=AXIS2_PLACEMENT_3D('',#38528,#30940,#30941);
#26186=AXIS2_PLACEMENT_3D('',#38529,#30942,#30943);
#26187=AXIS2_PLACEMENT_3D('',#38554,#30945,#30946);
#26188=AXIS2_PLACEMENT_3D('',#38557,#30948,#30949);
#26189=AXIS2_PLACEMENT_3D('',#38559,#30950,#30951);
#26190=AXIS2_PLACEMENT_3D('',#38576,#30952,#30953);
#26191=AXIS2_PLACEMENT_3D('',#38624,#30955,#30956);
#26192=AXIS2_PLACEMENT_3D('',#38672,#30958,#30959);
#26193=AXIS2_PLACEMENT_3D('',#38726,#30961,#30962);
#26194=AXIS2_PLACEMENT_3D('',#38774,#30964,#30965);
#26195=AXIS2_PLACEMENT_3D('',#38822,#30967,#30968);
#26196=AXIS2_PLACEMENT_3D('',#38873,#30970,#30971);
#26197=AXIS2_PLACEMENT_3D('',#38921,#30973,#30974);
#26198=AXIS2_PLACEMENT_3D('',#38936,#30976,#30977);
#26199=AXIS2_PLACEMENT_3D('',#38945,#30978,#30979);
#26200=AXIS2_PLACEMENT_3D('',#38970,#30981,#30982);
#26201=AXIS2_PLACEMENT_3D('',#38995,#30984,#30985);
#26202=AXIS2_PLACEMENT_3D('',#39019,#30987,#30988);
#26203=AXIS2_PLACEMENT_3D('',#39044,#30990,#30991);
#26204=AXIS2_PLACEMENT_3D('',#39069,#30993,#30994);
#26205=AXIS2_PLACEMENT_3D('',#39093,#30996,#30997);
#26206=AXIS2_PLACEMENT_3D('',#39458,#30999,#31000);
#26207=AXIS2_PLACEMENT_3D('',#39509,#31001,#31002);
#26208=AXIS2_PLACEMENT_3D('',#39510,#31003,#31004);
#26209=AXIS2_PLACEMENT_3D('',#39796,#31005,#31006);
#26210=AXIS2_PLACEMENT_3D('',#39797,#31007,#31008);
#26211=AXIS2_PLACEMENT_3D('',#39798,#31009,#31010);
#26212=AXIS2_PLACEMENT_3D('',#39802,#31012,#31013);
#26213=AXIS2_PLACEMENT_3D('',#39803,#31014,#31015);
#26214=AXIS2_PLACEMENT_3D('',#39806,#31017,#31018);
#26215=AXIS2_PLACEMENT_3D('',#39807,#31019,#31020);
#26216=AXIS2_PLACEMENT_3D('',#39810,#31022,#31023);
#26217=AXIS2_PLACEMENT_3D('',#39811,#31024,#31025);
#26218=AXIS2_PLACEMENT_3D('',#39821,#31026,#31027);
#26219=AXIS2_PLACEMENT_3D('',#39822,#31028,#31029);
#26220=AXIS2_PLACEMENT_3D('',#39832,#31030,#31031);
#26221=AXIS2_PLACEMENT_3D('',#39833,#31032,#31033);
#26222=AXIS2_PLACEMENT_3D('',#39843,#31034,#31035);
#26223=AXIS2_PLACEMENT_3D('',#39844,#31036,#31037);
#26224=AXIS2_PLACEMENT_3D('',#39854,#31038,#31039);
#26225=AXIS2_PLACEMENT_3D('',#39855,#31040,#31041);
#26226=AXIS2_PLACEMENT_3D('',#39865,#31042,#31043);
#26227=AXIS2_PLACEMENT_3D('',#39866,#31044,#31045);
#26228=AXIS2_PLACEMENT_3D('',#39873,#31046,#31047);
#26229=AXIS2_PLACEMENT_3D('',#39877,#31048,#31049);
#26230=AXIS2_PLACEMENT_3D('',#39892,#31054,#31055);
#26231=AXIS2_PLACEMENT_3D('',#39905,#31059,#31060);
#26232=AXIS2_PLACEMENT_3D('',#39918,#31064,#31065);
#26233=AXIS2_PLACEMENT_3D('',#39922,#31069,#31070);
#26234=AXIS2_PLACEMENT_3D('',#39934,#31073,#31074);
#26235=AXIS2_PLACEMENT_3D('',#39941,#31075,#31076);
#26236=AXIS2_PLACEMENT_3D('',#39945,#31077,#31078);
#26237=AXIS2_PLACEMENT_3D('',#39947,#31079,#31080);
#26238=AXIS2_PLACEMENT_3D('',#39951,#31081,#31082);
#26239=AXIS2_PLACEMENT_3D('',#39952,#31083,#31084);
#26240=AXIS2_PLACEMENT_3D('',#39953,#31085,#31086);
#26241=AXIS2_PLACEMENT_3D('',#39954,#31087,#31088);
#26242=AXIS2_PLACEMENT_3D('',#39955,#31089,#31090);
#26243=AXIS2_PLACEMENT_3D('',#39956,#31091,#31092);
#26244=AXIS2_PLACEMENT_3D('',#39957,#31093,#31094);
#26245=AXIS2_PLACEMENT_3D('',#39962,#31095,#31096);
#26246=AXIS2_PLACEMENT_3D('',#39963,#31097,#31098);
#26247=AXIS2_PLACEMENT_3D('',#39966,#31101,#31102);
#26248=AXIS2_PLACEMENT_3D('',#39968,#31103,#31104);
#26249=AXIS2_PLACEMENT_3D('',#39969,#31105,#31106);
#26250=AXIS2_PLACEMENT_3D('',#39971,#31108,#31109);
#26251=AXIS2_PLACEMENT_3D('',#39973,#31111,#31112);
#30940=DIRECTION('axis',(0.,0.,1.));
#30941=DIRECTION('refdir',(1.,0.,0.));
#30942=DIRECTION('center_axis',(0.,0.,1.));
#30943=DIRECTION('ref_axis',(1.,0.,0.));
#30944=DIRECTION('',(0.,0.,-1.));
#30945=DIRECTION('center_axis',(0.,0.,-1.));
#30946=DIRECTION('ref_axis',(1.,0.,0.));
#30947=DIRECTION('',(0.,0.,-1.));
#30948=DIRECTION('center_axis',(0.,0.,1.));
#30949=DIRECTION('ref_axis',(1.,0.,0.));
#30950=DIRECTION('center_axis',(0.,0.,-1.));
#30951=DIRECTION('ref_axis',(1.,0.,0.));
#30952=DIRECTION('center_axis',(0.,0.,1.));
#30953=DIRECTION('ref_axis',(1.,0.,0.));
#30954=DIRECTION('',(0.,0.,-1.));
#30955=DIRECTION('center_axis',(0.,0.,1.));
#30956=DIRECTION('ref_axis',(1.,0.,0.));
#30957=DIRECTION('',(0.,0.,-1.));
#30958=DIRECTION('center_axis',(0.,0.,1.));
#30959=DIRECTION('ref_axis',(1.,0.,0.));
#30960=DIRECTION('',(0.,0.,-1.));
#30961=DIRECTION('center_axis',(0.,0.,1.));
#30962=DIRECTION('ref_axis',(1.,0.,0.));
#30963=DIRECTION('',(0.,0.,-1.));
#30964=DIRECTION('center_axis',(0.,0.,1.));
#30965=DIRECTION('ref_axis',(1.,0.,0.));
#30966=DIRECTION('',(0.,0.,-1.));
#30967=DIRECTION('center_axis',(0.,0.,1.));
#30968=DIRECTION('ref_axis',(1.,0.,0.));
#30969=DIRECTION('',(0.,0.,-1.));
#30970=DIRECTION('center_axis',(0.,0.,1.));
#30971=DIRECTION('ref_axis',(1.,0.,0.));
#30972=DIRECTION('',(0.,0.,-1.));
#30973=DIRECTION('center_axis',(0.,0.,1.));
#30974=DIRECTION('ref_axis',(0.918748963007942,-0.394842174763325,0.));
#30975=DIRECTION('',(0.,0.,1.));
#30976=DIRECTION('center_axis',(0.,0.,1.));
#30977=DIRECTION('ref_axis',(1.,3.85997805270075E-14,0.));
#30978=DIRECTION('center_axis',(0.,0.,1.));
#30979=DIRECTION('ref_axis',(1.,3.85997805270075E-14,0.));
#30980=DIRECTION('',(0.,0.,1.));
#30981=DIRECTION('center_axis',(0.,0.,1.));
#30982=DIRECTION('ref_axis',(1.,3.85997805270075E-14,0.));
#30983=DIRECTION('',(0.,0.,1.));
#30984=DIRECTION('center_axis',(0.,0.,1.));
#30985=DIRECTION('ref_axis',(1.,3.85997805270075E-14,0.));
#30986=DIRECTION('',(0.,0.,1.));
#30987=DIRECTION('center_axis',(0.,0.,1.));
#30988=DIRECTION('ref_axis',(1.,3.85997805270075E-14,0.));
#30989=DIRECTION('',(0.,0.,1.));
#30990=DIRECTION('center_axis',(0.,0.,1.));
#30991=DIRECTION('ref_axis',(1.,3.85997805270075E-14,0.));
#30992=DIRECTION('',(0.,0.,1.));
#30993=DIRECTION('center_axis',(0.,0.,1.));
#30994=DIRECTION('ref_axis',(1.,3.85997805270075E-14,0.));
#30995=DIRECTION('',(0.,0.,1.));
#30996=DIRECTION('center_axis',(0.,0.,1.));
#30997=DIRECTION('ref_axis',(1.,3.85997805270075E-14,0.));
#30998=DIRECTION('',(0.,0.,1.));
#30999=DIRECTION('center_axis',(0.,0.,1.));
#31000=DIRECTION('ref_axis',(1.,0.,0.));
#31001=DIRECTION('center_axis',(0.,0.,-1.));
#31002=DIRECTION('ref_axis',(1.,3.85997805270075E-14,0.));
#31003=DIRECTION('center_axis',(0.,0.,1.));
#31004=DIRECTION('ref_axis',(-0.518977820445148,0.854787705741024,0.));
#31005=DIRECTION('center_axis',(0.,0.,1.));
#31006=DIRECTION('ref_axis',(1.,0.,0.));
#31007=DIRECTION('center_axis',(0.,0.,-1.));
#31008=DIRECTION('ref_axis',(1.,0.,0.));
#31009=DIRECTION('center_axis',(0.,0.,1.));
#31010=DIRECTION('ref_axis',(1.,0.,0.));
#31011=DIRECTION('',(-0.857167300702112,-1.04972719113862E-16,0.515038074910054));
#31012=DIRECTION('center_axis',(0.,0.,1.));
#31013=DIRECTION('ref_axis',(1.,0.,0.));
#31014=DIRECTION('center_axis',(0.,0.,1.));
#31015=DIRECTION('ref_axis',(1.,0.,0.));
#31016=DIRECTION('',(0.,0.,1.));
#31017=DIRECTION('center_axis',(0.,0.,1.));
#31018=DIRECTION('ref_axis',(1.,0.,0.));
#31019=DIRECTION('center_axis',(0.,0.,1.));
#31020=DIRECTION('ref_axis',(1.,0.,0.));
#31021=DIRECTION('',(-0.707106781186547,-8.65956056235493E-17,0.707106781186548));
#31022=DIRECTION('center_axis',(0.,0.,-1.));
#31023=DIRECTION('ref_axis',(1.,0.,0.));
#31024=DIRECTION('center_axis',(0.,0.,1.));
#31025=DIRECTION('ref_axis',(1.,0.,0.));
#31026=DIRECTION('center_axis',(0.,0.,-1.));
#31027=DIRECTION('ref_axis',(1.,0.,0.));
#31028=DIRECTION('center_axis',(0.,0.,1.));
#31029=DIRECTION('ref_axis',(1.,0.,0.));
#31030=DIRECTION('center_axis',(0.,0.,-1.));
#31031=DIRECTION('ref_axis',(1.,0.,0.));
#31032=DIRECTION('center_axis',(0.,0.,1.));
#31033=DIRECTION('ref_axis',(-1.,-1.22464679914735E-16,0.));
#31034=DIRECTION('center_axis',(0.,0.,-1.));
#31035=DIRECTION('ref_axis',(1.,0.,0.));
#31036=DIRECTION('center_axis',(0.,0.,1.));
#31037=DIRECTION('ref_axis',(1.,0.,0.));
#31038=DIRECTION('center_axis',(0.,0.,-1.));
#31039=DIRECTION('ref_axis',(1.,0.,0.));
#31040=DIRECTION('center_axis',(0.,0.,1.));
#31041=DIRECTION('ref_axis',(1.,0.,0.));
#31042=DIRECTION('center_axis',(0.,0.,-1.));
#31043=DIRECTION('ref_axis',(1.,0.,0.));
#31044=DIRECTION('center_axis',(0.,0.,1.));
#31045=DIRECTION('ref_axis',(1.,0.,0.));
#31046=DIRECTION('center_axis',(0.,0.,-1.));
#31047=DIRECTION('ref_axis',(1.,0.,0.));
#31048=DIRECTION('center_axis',(-1.92296268638356E-16,-1.,0.));
#31049=DIRECTION('ref_axis',(1.,-1.92296268638356E-16,0.));
#31050=DIRECTION('',(0.,0.,1.));
#31051=DIRECTION('',(1.,-1.92296268638356E-16,0.));
#31052=DIRECTION('',(0.,0.,1.));
#31053=DIRECTION('',(1.,-1.92296268638356E-16,0.));
#31054=DIRECTION('center_axis',(-0.866025403784439,-0.5,0.));
#31055=DIRECTION('ref_axis',(0.5,-0.866025403784439,0.));
#31056=DIRECTION('',(0.5,-0.866025403784439,0.));
#31057=DIRECTION('',(0.,0.,1.));
#31058=DIRECTION('',(0.5,-0.866025403784439,0.));
#31059=DIRECTION('center_axis',(-0.866025403784438,0.5,0.));
#31060=DIRECTION('ref_axis',(-0.5,-0.866025403784438,0.));
#31061=DIRECTION('',(-0.5,-0.866025403784438,0.));
#31062=DIRECTION('',(0.,0.,1.));
#31063=DIRECTION('',(-0.5,-0.866025403784438,0.));
#31064=DIRECTION('center_axis',(0.,0.,1.));
#31065=DIRECTION('ref_axis',(1.,0.,0.));
#31066=DIRECTION('',(0.5,0.866025403784439,0.));
#31067=DIRECTION('',(-1.,1.92296268638356E-16,0.));
#31068=DIRECTION('',(-0.5,0.866025403784439,0.));
#31069=DIRECTION('center_axis',(1.92296268638356E-16,1.,0.));
#31070=DIRECTION('ref_axis',(-1.,1.92296268638356E-16,0.));
#31071=DIRECTION('',(-1.,1.92296268638356E-16,0.));
#31072=DIRECTION('',(0.,0.,1.));
#31073=DIRECTION('center_axis',(0.,0.,-1.));
#31074=DIRECTION('ref_axis',(1.,0.,0.));
#31075=DIRECTION('center_axis',(0.,0.,1.));
#31076=DIRECTION('ref_axis',(1.,0.,0.));
#31077=DIRECTION('center_axis',(0.,0.,-1.));
#31078=DIRECTION('ref_axis',(1.,0.,0.));
#31079=DIRECTION('center_axis',(0.,0.,1.));
#31080=DIRECTION('ref_axis',(1.,0.,0.));
#31081=DIRECTION('center_axis',(0.,0.,-1.));
#31082=DIRECTION('ref_axis',(1.,0.,0.));
#31083=DIRECTION('center_axis',(0.,0.,1.));
#31084=DIRECTION('ref_axis',(1.,0.,0.));
#31085=DIRECTION('center_axis',(0.,0.,-1.));
#31086=DIRECTION('ref_axis',(-1.,-1.01064309961486E-15,0.));
#31087=DIRECTION('center_axis',(0.,0.,1.));
#31088=DIRECTION('ref_axis',(1.,0.,0.));
#31089=DIRECTION('center_axis',(0.,0.,-1.));
#31090=DIRECTION('ref_axis',(1.,0.,0.));
#31091=DIRECTION('center_axis',(0.,0.,1.));
#31092=DIRECTION('ref_axis',(1.,0.,0.));
#31093=DIRECTION('center_axis',(0.,0.,-1.));
#31094=DIRECTION('ref_axis',(1.,0.,0.));
#31095=DIRECTION('center_axis',(0.,0.,1.));
#31096=DIRECTION('ref_axis',(1.,0.,0.));
#31097=DIRECTION('center_axis',(0.866025403784439,-0.5,0.));
#31098=DIRECTION('ref_axis',(0.5,0.866025403784439,0.));
#31099=DIRECTION('',(0.,0.,1.));
#31100=DIRECTION('',(0.5,0.866025403784439,0.));
#31101=DIRECTION('center_axis',(0.,0.,-1.));
#31102=DIRECTION('ref_axis',(-1.,0.,0.));
#31103=DIRECTION('center_axis',(0.,0.,1.));
#31104=DIRECTION('ref_axis',(1.,0.,0.));
#31105=DIRECTION('center_axis',(0.,0.,1.));
#31106=DIRECTION('ref_axis',(1.,0.,0.));
#31107=DIRECTION('',(0.707106781186547,8.65956056235493E-17,-0.707106781186548));
#31108=DIRECTION('center_axis',(0.866025403784439,0.5,0.));
#31109=DIRECTION('ref_axis',(-0.5,0.866025403784439,0.));
#31110=DIRECTION('',(-0.5,0.866025403784439,0.));
#31111=DIRECTION('center_axis',(0.,0.,1.));
#31112=DIRECTION('ref_axis',(1.,0.,0.));
#38528=CARTESIAN_POINT('',(0.,0.,0.));
#38529=CARTESIAN_POINT('Origin',(0.,0.,-0.19));
#38530=CARTESIAN_POINT('',(-0.12155579423589,0.000100027207062599,-0.324010734985006));
#38531=CARTESIAN_POINT('',(-0.121567991859644,0.000104017427664388,-0.330489265014994));
#38532=CARTESIAN_POINT('',(-0.1215,-1.48794586096403E-17,-0.19));
#38533=CARTESIAN_POINT('',(-0.0374782951795791,-0.115758143579925,-0.36));
#38534=CARTESIAN_POINT('Ctrl Pts',(-0.12155579423589,0.000100027207062599,
-0.324010734985006));
#38535=CARTESIAN_POINT('Ctrl Pts',(-0.121620634124682,0.0074842758651267,
-0.32444665059017));
#38536=CARTESIAN_POINT('Ctrl Pts',(-0.121004234176155,0.0148576610554614,
-0.324882566195334));
#38537=CARTESIAN_POINT('Ctrl Pts',(-0.119667279374296,0.022097896271274,
-0.325318481800499));
#38538=CARTESIAN_POINT('Ctrl Pts',(-0.11243718511193,0.0612522364323941,
-0.327675862103401));
#38539=CARTESIAN_POINT('Ctrl Pts',(-0.0841343262472267,0.0965125801032592,
-0.330033242406302));
#38540=CARTESIAN_POINT('Ctrl Pts',(-0.0474717895588589,0.112047042615882,
-0.332390622709205));
#38541=CARTESIAN_POINT('Ctrl Pts',(-0.0108092528704911,0.127581505128506,
-0.334748003012107));
#38542=CARTESIAN_POINT('Ctrl Pts',(0.0342129616415417,0.123390086482887,
-0.337105383315009));
#38543=CARTESIAN_POINT('Ctrl Pts',(0.0673711970604704,0.101343025426172,
-0.339462763617911));
#38544=CARTESIAN_POINT('Ctrl Pts',(0.100529432479399,0.079295964369458,
-0.341820143920814));
#38545=CARTESIAN_POINT('Ctrl Pts',(0.121823688805224,0.0393932609016481,
-0.344177524223715));
#38546=CARTESIAN_POINT('Ctrl Pts',(0.121689461571731,-0.000417576977033936,
-0.346534904526618));
#38547=CARTESIAN_POINT('Ctrl Pts',(0.121555234338239,-0.0402284148557158,
-0.34889228482952));
#38548=CARTESIAN_POINT('Ctrl Pts',(0.0999925235454301,-0.0799473871452696,
-0.351249665132422));
#38549=CARTESIAN_POINT('Ctrl Pts',(0.0666859483039566,-0.101778801767896,
-0.353607045435324));
#38550=CARTESIAN_POINT('Ctrl Pts',(0.036578032614443,-0.121513595455792,
-0.355738030290216));
#38551=CARTESIAN_POINT('Ctrl Pts',(-0.00312637396201031,-0.126631583500994,
-0.357869015145108));
#38552=CARTESIAN_POINT('Ctrl Pts',(-0.0374782951795791,-0.115758143579925,
-0.36));
#38553=CARTESIAN_POINT('',(-0.1215,-1.48794586096403E-17,-0.36));
#38554=CARTESIAN_POINT('Origin',(0.,0.,-0.36));
#38555=CARTESIAN_POINT('',(-0.1215,-1.48794586096403E-17,-0.3835));
#38556=CARTESIAN_POINT('',(-0.1215,-1.48794586096403E-17,-0.19));
#38557=CARTESIAN_POINT('Origin',(0.,0.,-0.3835));
#38558=CARTESIAN_POINT('',(0.0677908815531582,-0.100829789141135,-0.36));
#38559=CARTESIAN_POINT('Origin',(0.,0.,-0.36));
#38560=CARTESIAN_POINT('Ctrl Pts',(0.0677908815531583,-0.100829789141135,
-0.36));
#38561=CARTESIAN_POINT('Ctrl Pts',(0.100979247033071,-0.07851625886049,
-0.357642619697098));
#38562=CARTESIAN_POINT('Ctrl Pts',(0.12202917251289,-0.0387425950814313,
-0.355285239394196));
#38563=CARTESIAN_POINT('Ctrl Pts',(0.121678176144516,0.00100886688157746,
-0.352927859091294));
#38564=CARTESIAN_POINT('Ctrl Pts',(0.121327179776142,0.0407603288445865,
-0.350570478788391));
#38565=CARTESIAN_POINT('Ctrl Pts',(0.0995752615595766,0.0804895889915456,
-0.348213098485489));
#38566=CARTESIAN_POINT('Ctrl Pts',(0.0661601753453354,0.102160099321753,
-0.345855718182587));
#38567=CARTESIAN_POINT('Ctrl Pts',(0.0327450891310943,0.123830609651961,
-0.343498337879685));
#38568=CARTESIAN_POINT('Ctrl Pts',(-0.012333165080822,0.127442370165417,
-0.341140957576783));
#38569=CARTESIAN_POINT('Ctrl Pts',(-0.0488096494985592,0.111460993500232,
-0.338783577273881));
#38570=CARTESIAN_POINT('Ctrl Pts',(-0.0852861339162964,0.0954796168350458,
-0.336426196970979));
#38571=CARTESIAN_POINT('Ctrl Pts',(-0.113160848539854,0.0599051029912176,
-0.334068816668076));
#38572=CARTESIAN_POINT('Ctrl Pts',(-0.11992145607908,0.0206722787223513,
-0.331711436365174));
#38573=CARTESIAN_POINT('Ctrl Pts',(-0.121089789820009,0.0138922619739541,
-0.331304045915114));
#38574=CARTESIAN_POINT('Ctrl Pts',(-0.12162755094405,0.00700298981783844,
-0.330896655465054));
#38575=CARTESIAN_POINT('Ctrl Pts',(-0.121567991859644,0.000104017427664388,
-0.330489265014994));
#38576=CARTESIAN_POINT('Origin',(0.,0.,-0.19));
#38577=CARTESIAN_POINT('',(-0.121316684751533,-2.98164701347942E-5,-0.279010734985006));
#38578=CARTESIAN_POINT('',(-0.1213134883411,-2.23347955230942E-5,-0.285489265014994));
#38579=CARTESIAN_POINT('',(-0.1215,-1.48794586096403E-17,-0.19));
#38580=CARTESIAN_POINT('Ctrl Pts',(-0.121316684751533,-2.98164701347942E-5,
-0.279010734985006));
#38581=CARTESIAN_POINT('Ctrl Pts',(-0.121267388452722,0.0219598511007976,
-0.280302368772757));
#38582=CARTESIAN_POINT('Ctrl Pts',(-0.115545772107405,0.0439734214389766,
-0.281594002560508));
#38583=CARTESIAN_POINT('Ctrl Pts',(-0.104309833231411,0.0626737375079338,
-0.282885636348259));
#38584=CARTESIAN_POINT('Ctrl Pts',(-0.0838029517592271,0.0968039663522564,
-0.285243016651162));
#38585=CARTESIAN_POINT('Ctrl Pts',(-0.0449276135031733,0.119897595955311,
-0.287600396954064));
#38586=CARTESIAN_POINT('Ctrl Pts',(-0.00514607383054742,0.1215814300281,
-0.289957777256966));
#38587=CARTESIAN_POINT('Ctrl Pts',(0.0346354658420782,0.123265264100889,
-0.292315157559868));
#38588=CARTESIAN_POINT('Ctrl Pts',(0.075323206931276,0.103539302643412,
-0.29467253786277));
#38589=CARTESIAN_POINT('Ctrl Pts',(0.0986407780548691,0.0712639068871239,
-0.297029918165672));
#38590=CARTESIAN_POINT('Ctrl Pts',(0.121958349178462,0.0389885111308361,
-0.299387298468575));
#38591=CARTESIAN_POINT('Ctrl Pts',(0.127905750336451,-0.00583631892426194,
-0.301744678771477));
#38592=CARTESIAN_POINT('Ctrl Pts',(0.113811504451575,-0.0430753921798633,
-0.304102059074379));
#38593=CARTESIAN_POINT('Ctrl Pts',(0.0997172585667,-0.0803144654354648,
-0.306459439377281));
#38594=CARTESIAN_POINT('Ctrl Pts',(0.0655813656389605,-0.109967781891569,
-0.308816819680183));
#38595=CARTESIAN_POINT('Ctrl Pts',(0.0267371682304334,-0.118716443260442,
-0.311174199983086));
#38596=CARTESIAN_POINT('Ctrl Pts',(-0.0121070291780935,-0.127465104629315,
-0.313531580285988));
#38597=CARTESIAN_POINT('Ctrl Pts',(-0.0556595310674075,-0.115309110910955,
-0.315888960588889));
#38598=CARTESIAN_POINT('Ctrl Pts',(-0.0843571171820498,-0.0877069457260886,
-0.318246340891792));
#38599=CARTESIAN_POINT('Ctrl Pts',(-0.107748081534174,-0.0652088422514121,
-0.32016780558953));
#38600=CARTESIAN_POINT('Ctrl Pts',(-0.121269987635155,-0.0324488720470692,
-0.322089270287268));
#38601=CARTESIAN_POINT('Ctrl Pts',(-0.12155579423589,0.000100027207062599,
-0.324010734985006));
#38602=CARTESIAN_POINT('Ctrl Pts',(-0.121567991859644,0.000104017427664388,
-0.330489265014994));
#38603=CARTESIAN_POINT('Ctrl Pts',(-0.121282910041409,-0.0329181757874598,
-0.328539275162152));
#38604=CARTESIAN_POINT('Ctrl Pts',(-0.107312657409089,-0.0661626105376077,
-0.32658928530931));
#38605=CARTESIAN_POINT('Ctrl Pts',(-0.0833038297687421,-0.0887116572214725,
-0.324639295456468));
#38606=CARTESIAN_POINT('Ctrl Pts',(-0.0542790954642872,-0.115971634202525,
-0.322281915153566));
#38607=CARTESIAN_POINT('Ctrl Pts',(-0.0105831264004852,-0.127600453470727,
-0.319924534850663));
#38608=CARTESIAN_POINT('Ctrl Pts',(0.0281540805652533,-0.118386890783788,
-0.317567154547761));
#38609=CARTESIAN_POINT('Ctrl Pts',(0.0668912875309918,-0.10917332809685,
-0.315209774244859));
#38610=CARTESIAN_POINT('Ctrl Pts',(0.100669732398667,-0.0791173834547723,
-0.312852393941957));
#38611=CARTESIAN_POINT('Ctrl Pts',(0.114317861247938,-0.0417133069274287,
-0.310495013639055));
#38612=CARTESIAN_POINT('Ctrl Pts',(0.127965990097209,-0.00430923040008524,
-0.308137633336153));
#38613=CARTESIAN_POINT('Ctrl Pts',(0.121483802928076,0.0404429780125239,
-0.30578025303325));
#38614=CARTESIAN_POINT('Ctrl Pts',(0.0977823489008379,0.0724378514980737,
-0.303422872730348));
#38615=CARTESIAN_POINT('Ctrl Pts',(0.0740808948735994,0.104432724983624,
-0.301065492427446));
#38616=CARTESIAN_POINT('Ctrl Pts',(0.0331601739882546,0.123670263542114,
-0.298708112124544));
#38617=CARTESIAN_POINT('Ctrl Pts',(-0.00659845091904251,0.121511023160459,
-0.296350731821642));
#38618=CARTESIAN_POINT('Ctrl Pts',(-0.0463570758263398,0.119351782778803,
-0.29399335151874));
#38619=CARTESIAN_POINT('Ctrl Pts',(-0.0849536047555895,0.095795763457001,
-0.291635971215837));
#38620=CARTESIAN_POINT('Ctrl Pts',(-0.105051198646726,0.0614230580704297,
-0.289278590912935));
#38621=CARTESIAN_POINT('Ctrl Pts',(-0.115819696333789,0.0430058086992691,
-0.288015482280288));
#38622=CARTESIAN_POINT('Ctrl Pts',(-0.12127728535159,0.0214831680352748,
-0.286752373647641));
#38623=CARTESIAN_POINT('Ctrl Pts',(-0.1213134883411,-2.23347955230942E-5,
-0.285489265014994));
#38624=CARTESIAN_POINT('Origin',(0.,0.,-0.19));
#38625=CARTESIAN_POINT('',(-0.121652121442684,-5.9196348637991E-5,-0.234010734985006));
#38626=CARTESIAN_POINT('',(-0.121642193667188,-6.59388428620122E-5,-0.240489265014994));
#38627=CARTESIAN_POINT('',(-0.1215,-1.48794586096403E-17,-0.19));
#38628=CARTESIAN_POINT('Ctrl Pts',(-0.121652121442684,-5.9196348637991E-5,
-0.234010734985006));
#38629=CARTESIAN_POINT('Ctrl Pts',(-0.121432098146049,0.0362408929853419,
-0.236158086955344));
#38630=CARTESIAN_POINT('Ctrl Pts',(-0.104092725076878,0.0727236629989947,
-0.238305438925682));
#38631=CARTESIAN_POINT('Ctrl Pts',(-0.0756934135126743,0.0952840140834343,
-0.240452790896021));
#38632=CARTESIAN_POINT('Ctrl Pts',(-0.0445164203498382,0.12005094936356,
-0.242810171198923));
#38633=CARTESIAN_POINT('Ctrl Pts',(-1.01824319385865E-5,0.128038828451523,
-0.245167551501825));
#38634=CARTESIAN_POINT('Ctrl Pts',(0.0378337200468045,0.11565961062334,
-0.247524931804727));
#38635=CARTESIAN_POINT('Ctrl Pts',(0.0756776225255475,0.103280392795157,
-0.249882312107629));
#38636=CARTESIAN_POINT('Ctrl Pts',(0.106859189565134,0.0705340780508277,
-0.252239692410531));
#38637=CARTESIAN_POINT('Ctrl Pts',(0.117372096756334,0.032129847839524,
-0.254597072713433));
#38638=CARTESIAN_POINT('Ctrl Pts',(0.127885003947534,-0.00627438237177978,
-0.256954453016336));
#38639=CARTESIAN_POINT('Ctrl Pts',(0.117729251290347,-0.0503365280500584,
-0.259311833319238));
#38640=CARTESIAN_POINT('Ctrl Pts',(0.0914666612543121,-0.0802644782613266,
-0.26166921362214));
#38641=CARTESIAN_POINT('Ctrl Pts',(0.0652040712182769,-0.110192428472595,
-0.264026593925042));
#38642=CARTESIAN_POINT('Ctrl Pts',(0.0228346438033933,-0.125986183216853,
-0.266383974227944));
#38643=CARTESIAN_POINT('Ctrl Pts',(-0.0166098666488376,-0.120551428846724,
-0.268741354530847));
#38644=CARTESIAN_POINT('Ctrl Pts',(-0.0560543771010683,-0.115116674476596,
-0.271098734833749));
#38645=CARTESIAN_POINT('Ctrl Pts',(-0.0925739705906463,-0.0884534109920819,
-0.273456115136651));
#38646=CARTESIAN_POINT('Ctrl Pts',(-0.109764554991278,-0.0525383652070299,
-0.275813495439553));
#38647=CARTESIAN_POINT('Ctrl Pts',(-0.117536235019243,-0.0363015557114269,
-0.276879241954704));
#38648=CARTESIAN_POINT('Ctrl Pts',(-0.121357359871034,-0.0181738227707557,
-0.277944988469855));
#38649=CARTESIAN_POINT('Ctrl Pts',(-0.121316684751533,-2.98164701347942E-5,
-0.279010734985006));
#38650=CARTESIAN_POINT('Ctrl Pts',(-0.1213134883411,-2.23347955230942E-5,
-0.285489265014994));
#38651=CARTESIAN_POINT('Ctrl Pts',(-0.121344852156353,-0.0186532441995837,
-0.284394993344739));
#38652=CARTESIAN_POINT('Ctrl Pts',(-0.117307295164673,-0.0372712911205606,
-0.283300721674484));
#38653=CARTESIAN_POINT('Ctrl Pts',(-0.109128983929891,-0.0538461772364694,
-0.282206450004229));
#38654=CARTESIAN_POINT('Ctrl Pts',(-0.0915105164688954,-0.0895533157054566,
-0.279849069701327));
#38655=CARTESIAN_POINT('Ctrl Pts',(-0.0546749226938819,-0.11577820119209,
-0.277491689398425));
#38656=CARTESIAN_POINT('Ctrl Pts',(-0.0151682872483324,-0.12074124246499,
-0.275134309095522));
#38657=CARTESIAN_POINT('Ctrl Pts',(0.0243383481972172,-0.12570428373789,
-0.27277692879262));
#38658=CARTESIAN_POINT('Ctrl Pts',(0.0665160253133027,-0.109405480797056,
-0.270419548489718));
#38659=CARTESIAN_POINT('Ctrl Pts',(0.0924191474222124,-0.0791658908688873,
-0.268062168186816));
#38660=CARTESIAN_POINT('Ctrl Pts',(0.118322269531122,-0.048926300940719,
-0.265704787883913));
#38661=CARTESIAN_POINT('Ctrl Pts',(0.127950836632856,-0.00474592402521655,
-0.263347407581011));
#38662=CARTESIAN_POINT('Ctrl Pts',(0.116979816901966,0.0335299595321455,
-0.260990027278109));
#38663=CARTESIAN_POINT('Ctrl Pts',(0.106008797171075,0.0718058430895075,
-0.258632646975207));
#38664=CARTESIAN_POINT('Ctrl Pts',(0.0744381906075608,0.104177233288729,
-0.256275266672305));
#38665=CARTESIAN_POINT('Ctrl Pts',(0.0364490799724483,0.116103391967299,
-0.253917886369403));
#38666=CARTESIAN_POINT('Ctrl Pts',(-0.0015400306626643,0.128029550645869,
-0.2515605060665));
#38667=CARTESIAN_POINT('Ctrl Pts',(-0.0459476453693751,0.119510477803787,
-0.249203125763598));
#38668=CARTESIAN_POINT('Ctrl Pts',(-0.0768264879290973,0.0943728019139746,
-0.246845745460696));
#38669=CARTESIAN_POINT('Ctrl Pts',(-0.104580567132348,0.0717789159455437,
-0.244726918645462));
#38670=CARTESIAN_POINT('Ctrl Pts',(-0.121405405335243,0.0357596639627758,
-0.242608091830228));
#38671=CARTESIAN_POINT('Ctrl Pts',(-0.121642193667188,-6.59388428620122E-5,
-0.240489265014994));
#38672=CARTESIAN_POINT('Origin',(0.,0.,-0.19));
#38673=CARTESIAN_POINT('',(-0.121452836205038,0.000103164027536851,-0.189010734985006));
#38674=CARTESIAN_POINT('',(-0.121466423015182,0.000104460321887741,-0.195489265014994));
#38675=CARTESIAN_POINT('',(-0.1215,-1.48794586096403E-17,-0.19));
#38676=CARTESIAN_POINT('Ctrl Pts',(-0.121452836205038,0.000103164027536851,
-0.189010734985006));
#38677=CARTESIAN_POINT('Ctrl Pts',(-0.121544980016008,0.0110647321231586,
-0.189656424835029));
#38678=CARTESIAN_POINT('Ctrl Pts',(-0.120180324762459,0.0220037716634773,
-0.190302114685052));
#38679=CARTESIAN_POINT('Ctrl Pts',(-0.117266460944003,0.0325132779165323,
-0.190947804535075));
#38680=CARTESIAN_POINT('Ctrl Pts',(-0.106628094597184,0.0708829425988793,
-0.193305184837977));
#38681=CARTESIAN_POINT('Ctrl Pts',(-0.075339670468586,0.103527175985459,
-0.19566256514088));
#38682=CARTESIAN_POINT('Ctrl Pts',(-0.0374555115366707,0.115782644476787,
-0.198019945443782));
#38683=CARTESIAN_POINT('Ctrl Pts',(0.000428647395244536,0.128038112968116,
-0.200377325746684));
#38684=CARTESIAN_POINT('Ctrl Pts',(0.0449085411304768,0.119904816564194,
-0.202734706049586));
#38685=CARTESIAN_POINT('Ctrl Pts',(0.0760044228399103,0.09503611844497,
-0.205092086352488));
#38686=CARTESIAN_POINT('Ctrl Pts',(0.107100304549344,0.0701674203257461,
-0.20744946665539));
#38687=CARTESIAN_POINT('Ctrl Pts',(0.124812174232979,0.0285633204912204,
-0.209806846958292));
#38688=CARTESIAN_POINT('Ctrl Pts',(0.121184107483162,-0.0110882007938326,
-0.212164227261195));
#38689=CARTESIAN_POINT('Ctrl Pts',(0.117556040733344,-0.0507397220788855,
-0.214521607564097));
#38690=CARTESIAN_POINT('Ctrl Pts',(0.0925880375500753,-0.0884386648144661,
-0.216878987866999));
#38691=CARTESIAN_POINT('Ctrl Pts',(0.0574953761353696,-0.107251190394802,
-0.219236368169901));
#38692=CARTESIAN_POINT('Ctrl Pts',(0.0224027147206637,-0.126063715975137,
-0.221593748472803));
#38693=CARTESIAN_POINT('Ctrl Pts',(-0.0228146049254789,-0.125989824400228,
-0.223951128775705));
#38694=CARTESIAN_POINT('Ctrl Pts',(-0.057845594568456,-0.107062707165432,
-0.226308509078608));
#38695=CARTESIAN_POINT('Ctrl Pts',(-0.0928765842114331,-0.0881355899306356,
-0.22866588938151));
#38696=CARTESIAN_POINT('Ctrl Pts',(-0.117721243851244,-0.0503552470359518,
-0.231023269684412));
#38697=CARTESIAN_POINT('Ctrl Pts',(-0.121219699467264,-0.0106920798524657,
-0.233380649987314));
#38698=CARTESIAN_POINT('Ctrl Pts',(-0.121531390711429,-0.00715833145493331,
-0.233590678319878));
#38699=CARTESIAN_POINT('Ctrl Pts',(-0.121673641494709,-0.00360963770154739,
-0.233800706652442));
#38700=CARTESIAN_POINT('Ctrl Pts',(-0.121652121442684,-5.9196348637991E-5,
-0.234010734985006));
#38701=CARTESIAN_POINT('Ctrl Pts',(-0.121642193667188,-6.59388428620122E-5,
-0.240489265014994));
#38702=CARTESIAN_POINT('Ctrl Pts',(-0.121668853081737,-0.00409945514332142,
-0.240250711527326));
#38703=CARTESIAN_POINT('Ctrl Pts',(-0.121485243156111,-0.00813051675591712,
-0.240012158039658));
#38704=CARTESIAN_POINT('Ctrl Pts',(-0.121083287896919,-0.0121396872446064,
-0.23977360455199));
#38705=CARTESIAN_POINT('Ctrl Pts',(-0.117111174892285,-0.0517582215758337,
-0.237416224249088));
#38706=CARTESIAN_POINT('Ctrl Pts',(-0.0918168784702831,-0.0892390113007461,
-0.235058843946185));
#38707=CARTESIAN_POINT('Ctrl Pts',(-0.0565622442669608,-0.107746214874363,
-0.232701463643283));
#38708=CARTESIAN_POINT('Ctrl Pts',(-0.0213076100636385,-0.12625341844798,
-0.230344083340381));
#38709=CARTESIAN_POINT('Ctrl Pts',(0.0239073619210042,-0.125787035870301,
-0.227986703037479));
#38710=CARTESIAN_POINT('Ctrl Pts',(0.058772738544517,-0.106556556759136,
-0.225629322734577));
#38711=CARTESIAN_POINT('Ctrl Pts',(0.0936381151680299,-0.0873260776479714,
-0.223271942431675));
#38712=CARTESIAN_POINT('Ctrl Pts',(0.118153896430413,-0.0493315020033205,
-0.220914562128773));
#38713=CARTESIAN_POINT('Ctrl Pts',(0.121307935605703,-0.00963946391216232,
-0.21855718182587));
#38714=CARTESIAN_POINT('Ctrl Pts',(0.124461974780992,0.0300525741789959,
-0.216199801522968));
#38715=CARTESIAN_POINT('Ctrl Pts',(0.106254271869187,0.0714420747166612,
-0.213842421220066));
#38716=CARTESIAN_POINT('Ctrl Pts',(0.0748634727914798,0.0959374531295166,
-0.211485040917164));
#38717=CARTESIAN_POINT('Ctrl Pts',(0.0434726737137725,0.120432831542372,
-0.209127660614262));
#38718=CARTESIAN_POINT('Ctrl Pts',(-0.00110122152983763,0.128034087830417,
-0.20677028031136));
#38719=CARTESIAN_POINT('Ctrl Pts',(-0.0388362420289081,0.115326843441258,
-0.204412900008457));
#38720=CARTESIAN_POINT('Ctrl Pts',(-0.0765712625279784,0.1026195990521,
-0.202055519705555));
#38721=CARTESIAN_POINT('Ctrl Pts',(-0.107467408282509,0.0696038539857373,
-0.199698139402653));
#38722=CARTESIAN_POINT('Ctrl Pts',(-0.117646562232706,0.0311098198818689,
-0.197340759099751));
#38723=CARTESIAN_POINT('Ctrl Pts',(-0.120311475668384,0.021032040414268,
-0.196723594404832));
#38724=CARTESIAN_POINT('Ctrl Pts',(-0.121556450581511,0.0105787800990859,
-0.196106429709913));
#38725=CARTESIAN_POINT('Ctrl Pts',(-0.121466423015182,0.000104460321887741,
-0.195489265014994));
#38726=CARTESIAN_POINT('Origin',(0.,0.,-0.19));
#38727=CARTESIAN_POINT('',(-0.121366189046343,-7.72277758326612E-5,-0.144010734985006));
#38728=CARTESIAN_POINT('',(-0.121356940814226,-7.17826249269161E-5,-0.150489265014994));
#38729=CARTESIAN_POINT('',(-0.1215,-1.48794586096403E-17,-0.19));
#38730=CARTESIAN_POINT('Ctrl Pts',(-0.121366189046343,-7.72277758326612E-5,
-0.144010734985006));
#38731=CARTESIAN_POINT('Ctrl Pts',(-0.121214006322019,0.0254575835671733,
-0.145512143017616));
#38732=CARTESIAN_POINT('Ctrl Pts',(-0.113325331544467,0.0510784255672011,
-0.147013551050226));
#38733=CARTESIAN_POINT('Ctrl Pts',(-0.0984073400571069,0.0715858330918497,
-0.148514959082836));
#38734=CARTESIAN_POINT('Ctrl Pts',(-0.0749844073650329,0.10378478068783,
-0.150872339385738));
#38735=CARTESIAN_POINT('Ctrl Pts',(-0.0342324172038069,0.123377808882716,
-0.15322971968864));
#38736=CARTESIAN_POINT('Ctrl Pts',(0.00554340599624446,0.121564002764019,
-0.155587099991543));
#38737=CARTESIAN_POINT('Ctrl Pts',(0.0453192291962959,0.119750196645322,
-0.157944480294445));
#38738=CARTESIAN_POINT('Ctrl Pts',(0.0841188854351726,0.0965295562130407,
-0.160301860597347));
#38739=CARTESIAN_POINT('Ctrl Pts',(0.104514111104929,0.0623324689329835,
-0.162659240900249));
#38740=CARTESIAN_POINT('Ctrl Pts',(0.124909336774685,0.0281353816529263,
-0.165016621203151));
#38741=CARTESIAN_POINT('Ctrl Pts',(0.126900131875321,-0.0170381524749071,
-0.167374001506053));
#38742=CARTESIAN_POINT('Ctrl Pts',(0.109592259115638,-0.0528968131577431,
-0.169731381808956));
#38743=CARTESIAN_POINT('Ctrl Pts',(0.0922843863559539,-0.0887554738405791,
-0.172088762111858));
#38744=CARTESIAN_POINT('Ctrl Pts',(0.0556778457359505,-0.115299261078418,
-0.17444614241476));
#38745=CARTESIAN_POINT('Ctrl Pts',(0.0162157838364738,-0.120605076431635,
-0.176803522717662));
#38746=CARTESIAN_POINT('Ctrl Pts',(-0.0232462780630026,-0.125910891784852,
-0.179160903020564));
#38747=CARTESIAN_POINT('Ctrl Pts',(-0.0655638612419521,-0.109978735253448,
-0.181518283323466));
#38748=CARTESIAN_POINT('Ctrl Pts',(-0.0917284985489071,-0.0799651089986894,
-0.183875663626369));
#38749=CARTESIAN_POINT('Ctrl Pts',(-0.110726604126622,-0.0581722580728937,
-0.185587354079248));
#38750=CARTESIAN_POINT('Ctrl Pts',(-0.121208567719907,-0.0289553870046511,
-0.187299044532127));
#38751=CARTESIAN_POINT('Ctrl Pts',(-0.121452836205038,0.000103164027536851,
-0.189010734985006));
#38752=CARTESIAN_POINT('Ctrl Pts',(-0.121466423015182,0.000104460321887741,
-0.195489265014994));
#38753=CARTESIAN_POINT('Ctrl Pts',(-0.121212572823547,-0.0294299166594152,
-0.193749049407011));
#38754=CARTESIAN_POINT('Ctrl Pts',(-0.110344552537344,-0.0591317305671495,
-0.192008833799028));
#38755=CARTESIAN_POINT('Ctrl Pts',(-0.0907664982302483,-0.081055396453563,
-0.190268618191044));
#38756=CARTESIAN_POINT('Ctrl Pts',(-0.0642451181317306,-0.110754255543751,
-0.187911237888142));
#38757=CARTESIAN_POINT('Ctrl Pts',(-0.0217401957888325,-0.126179650582752,
-0.18555385758524));
#38758=CARTESIAN_POINT('Ctrl Pts',(0.0176556515372683,-0.120402709563575,
-0.183196477282338));
#38759=CARTESIAN_POINT('Ctrl Pts',(0.057051498863369,-0.114625768544397,
-0.180839096979436));
#38760=CARTESIAN_POINT('Ctrl Pts',(0.0933382711726726,-0.087646491467041,
-0.178481716676534));
#38761=CARTESIAN_POINT('Ctrl Pts',(0.110216457309932,-0.0515835927033183,
-0.176124336373631));
#38762=CARTESIAN_POINT('Ctrl Pts',(0.127094643447192,-0.0155206939395955,
-0.173766956070729));
#38763=CARTESIAN_POINT('Ctrl Pts',(0.124564243412408,0.0296258265104934,
-0.171409575767827));
#38764=CARTESIAN_POINT('Ctrl Pts',(0.103761877546585,0.06357678244565,-0.169052195464925));
#38765=CARTESIAN_POINT('Ctrl Pts',(0.0829595116807615,0.0975277383808065,
-0.166694815162023));
#38766=CARTESIAN_POINT('Ctrl Pts',(0.0438851799838995,0.12028312980103,
-0.164337434859121));
#38767=CARTESIAN_POINT('Ctrl Pts',(0.00409052634720552,0.121621552759611,
-0.161980054556218));
#38768=CARTESIAN_POINT('Ctrl Pts',(-0.0357041272894885,0.122959975718192,
-0.159622674253316));
#38769=CARTESIAN_POINT('Ctrl Pts',(-0.0762191028660145,0.102881430215129,
-0.157265293950414));
#38770=CARTESIAN_POINT('Ctrl Pts',(-0.0992556394140983,0.0704049184341864,
-0.154907913647512));
#38771=CARTESIAN_POINT('Ctrl Pts',(-0.113648785991654,0.0501137087110959,
-0.153435030770006));
#38772=CARTESIAN_POINT('Ctrl Pts',(-0.121218863464572,0.0249826971880121,
-0.1519621478925));
#38773=CARTESIAN_POINT('Ctrl Pts',(-0.121356940814226,-7.17826249269161E-5,
-0.150489265014994));
#38774=CARTESIAN_POINT('Origin',(0.,0.,-0.19));
#38775=CARTESIAN_POINT('',(-0.121690333780732,-6.67349754346347E-8,-0.0990107349850059));
#38776=CARTESIAN_POINT('',(-0.121689496210452,-8.68452866517571E-6,-0.105489265014994));
#38777=CARTESIAN_POINT('',(-0.1215,-1.48794586096403E-17,-0.19));
#38778=CARTESIAN_POINT('Ctrl Pts',(-0.121690333780732,-6.67349754346347E-8,
-0.0990107349850059));
#38779=CARTESIAN_POINT('Ctrl Pts',(-0.121689956805147,0.0398128076349811,
-0.101367861200203));
#38780=CARTESIAN_POINT('Ctrl Pts',(-0.100266142222434,0.0796260065197837,
-0.1037249874154));
#38781=CARTESIAN_POINT('Ctrl Pts',(-0.0670395400323943,0.101559020964777,
-0.106082113630597));
#38782=CARTESIAN_POINT('Ctrl Pts',(-0.0338093561626619,0.123494399691016,
-0.108439493933499));
#38783=CARTESIAN_POINT('Ctrl Pts',(0.011226160027391,0.127545738961227,
-0.110796874236402));
#38784=CARTESIAN_POINT('Ctrl Pts',(0.0478376930952209,0.111893215660743,
-0.113154254539304));
#38785=CARTESIAN_POINT('Ctrl Pts',(0.0844492261630509,0.0962406923602585,
-0.115511634842206));
#38786=CARTESIAN_POINT('Ctrl Pts',(0.112636776108658,0.0608843064890792,
-0.117869015145108));
#38787=CARTESIAN_POINT('Ctrl Pts',(0.119738884453224,0.0217056621430117,
-0.12022639544801));
#38788=CARTESIAN_POINT('Ctrl Pts',(0.126840992797791,-0.0174729822030555,
-0.122583775750912));
#38789=CARTESIAN_POINT('Ctrl Pts',(0.112857659541317,-0.0604738850240109,
-0.124941156053815));
#38790=CARTESIAN_POINT('Ctrl Pts',(0.0840700051746493,-0.0879816465636836,
-0.127298536356717));
#38791=CARTESIAN_POINT('Ctrl Pts',(0.0552823508079815,-0.115489408103357,
-0.129655916659619));
#38792=CARTESIAN_POINT('Ctrl Pts',(0.0116903753311198,-0.127504028361747,
-0.132013296962521));
#38793=CARTESIAN_POINT('Ctrl Pts',(-0.0271250162488584,-0.118628705137298,
-0.134370677265423));
#38794=CARTESIAN_POINT('Ctrl Pts',(-0.0659404078288361,-0.109753381912849,
-0.136728057568325));
#38795=CARTESIAN_POINT('Ctrl Pts',(-0.0999792155119305,-0.079988115205563,
-0.139085437871228));
#38796=CARTESIAN_POINT('Ctrl Pts',(-0.113951681742017,-0.0427030483533834,
-0.14144281817413));
#38797=CARTESIAN_POINT('Ctrl Pts',(-0.11902512857867,-0.0291647222368194,
-0.142298790444422));
#38798=CARTESIAN_POINT('Ctrl Pts',(-0.121452950399159,-0.014634956229408,
-0.143154762714714));
#38799=CARTESIAN_POINT('Ctrl Pts',(-0.121366189046343,-7.72277758326612E-5,
-0.144010734985006));
#38800=CARTESIAN_POINT('Ctrl Pts',(-0.121356940814226,-7.17826249269161E-5,
-0.150489265014994));
#38801=CARTESIAN_POINT('Ctrl Pts',(-0.121439859192964,-0.0151175294576353,
-0.149604767589598));
#38802=CARTESIAN_POINT('Ctrl Pts',(-0.118842607042299,-0.0301356769858909,
-0.148720270164202));
#38803=CARTESIAN_POINT('Ctrl Pts',(-0.113433312185074,-0.044061527265631,
-0.147835772738805));
#38804=CARTESIAN_POINT('Ctrl Pts',(-0.0990163508883235,-0.0811769831256851,
-0.145478392435903));
#38805=CARTESIAN_POINT('Ctrl Pts',(-0.0646243307751811,-0.110533416786971,
-0.143121012133001));
#38806=CARTESIAN_POINT('Ctrl Pts',(-0.0257056668506945,-0.118944328174207,
-0.140763631830099));
#38807=CARTESIAN_POINT('Ctrl Pts',(0.0132129970737924,-0.127355239561444,
-0.138406251527197));
#38808=CARTESIAN_POINT('Ctrl Pts',(0.0566583048096238,-0.11482062867463,
-0.136048871224295));
#38809=CARTESIAN_POINT('Ctrl Pts',(0.0851152312342714,-0.0869708680151885,
-0.133691490921392));
#38810=CARTESIAN_POINT('Ctrl Pts',(0.113572157658919,-0.0591211073557473,
-0.13133411061849));
#38811=CARTESIAN_POINT('Ctrl Pts',(0.127040702772383,-0.0159561969236791,
-0.128976730315588));
#38812=CARTESIAN_POINT('Ctrl Pts',(0.119470984035321,0.0231347893671651,
-0.126619350012686));
#38813=CARTESIAN_POINT('Ctrl Pts',(0.11190126529826,0.0622257756580095,
-0.124261969709784));
#38814=CARTESIAN_POINT('Ctrl Pts',(0.0832932827106712,0.0972428378076296,
-0.121904589406882));
#38815=CARTESIAN_POINT('Ctrl Pts',(0.0464973428307525,0.112456799234482,
-0.11954720910398));
#38816=CARTESIAN_POINT('Ctrl Pts',(0.00970140295083383,0.127670760661335,
-0.117189828801077));
#38817=CARTESIAN_POINT('Ctrl Pts',(-0.035282494221415,0.12308162136542,
-0.114832448498175));
#38818=CARTESIAN_POINT('Ctrl Pts',(-0.0682482114436531,0.100750761441342,
-0.112475068195273));
#38819=CARTESIAN_POINT('Ctrl Pts',(-0.100811478378532,0.0786925199145164,
-0.11014646713518));
#38820=CARTESIAN_POINT('Ctrl Pts',(-0.121648213577836,0.0393231005841258,
-0.107817866075087));
#38821=CARTESIAN_POINT('Ctrl Pts',(-0.121689496210452,-8.6845286651757E-6,
-0.105489265014994));
#38822=CARTESIAN_POINT('Origin',(0.,0.,-0.19));
#38823=CARTESIAN_POINT('',(-0.121366197770921,7.70029837308187E-5,-0.0540107349850059));
#38824=CARTESIAN_POINT('',(-0.121376290077639,8.23099624828544E-5,-0.060489265014994));
#38825=CARTESIAN_POINT('',(-0.1215,-1.48794586096403E-17,-0.19));
#38826=CARTESIAN_POINT('Ctrl Pts',(-0.121366197770921,7.70029837308187E-5,
-0.0540107349850059));
#38827=CARTESIAN_POINT('Ctrl Pts',(-0.121453181762923,0.0146263535592494,
-0.0548661990798879));
#38828=CARTESIAN_POINT('Ctrl Pts',(-0.119028488418249,0.0291477473845937,
-0.0557216631747699));
#38829=CARTESIAN_POINT('Ctrl Pts',(-0.113961010341666,0.042679265103465,
-0.0565771272696519));
#38830=CARTESIAN_POINT('Ctrl Pts',(-0.0999966919388308,0.0799677188558563,
-0.0589345075725541));
#38831=CARTESIAN_POINT('Ctrl Pts',(-0.0659637531736886,0.1097393107365,
-0.0612918878754562));
#38832=CARTESIAN_POINT('Ctrl Pts',(-0.0271501406182937,0.118622678817329,
-0.0636492681783583));
#38833=CARTESIAN_POINT('Ctrl Pts',(0.0116634719371012,0.127506046898158,
-0.0660066484812605));
#38834=CARTESIAN_POINT('Ctrl Pts',(0.0552577582827487,0.115501191179173,
-0.0683640287841626));
#38835=CARTESIAN_POINT('Ctrl Pts',(0.0840512087018202,0.0879996720036106,
-0.0707214090870648));
#38836=CARTESIAN_POINT('Ctrl Pts',(0.112844659120892,0.0604981528280479,
-0.0730787893899669));
#38837=CARTESIAN_POINT('Ctrl Pts',(0.126837273613388,0.0174999701959076,
-0.0754361696928691));
#38838=CARTESIAN_POINT('Ctrl Pts',(0.119743536518744,-0.0216802440500727,
-0.0777935499957713));
#38839=CARTESIAN_POINT('Ctrl Pts',(0.112649799424101,-0.0608604582960528,
-0.0801509302986735));
#38840=CARTESIAN_POINT('Ctrl Pts',(0.0844697107423188,-0.096222704155873,
-0.0825083106015756));
#38841=CARTESIAN_POINT('Ctrl Pts',(0.0478614929616094,-0.111882991089053,
-0.0848656909044778));
#38842=CARTESIAN_POINT('Ctrl Pts',(0.0112532751809,-0.127543278022233,-0.0872230712073799));
#38843=CARTESIAN_POINT('Ctrl Pts',(-0.0337830716987367,-0.123501606028772,
-0.0895804515102821));
#38844=CARTESIAN_POINT('Ctrl Pts',(-0.0670179132089846,-0.10157331338049,
-0.0919378318131843));
#38845=CARTESIAN_POINT('Ctrl Pts',(-0.100256336900943,-0.0796426572147265,
-0.0942954662037915));
#38846=CARTESIAN_POINT('Ctrl Pts',(-0.121690710837589,-0.0398215244059149,
-0.0966531005943987));
#38847=CARTESIAN_POINT('Ctrl Pts',(-0.121690333780732,-6.67349754346347E-8,
-0.0990107349850059));
#38848=CARTESIAN_POINT('Ctrl Pts',(-0.121689496210452,-8.6845286651757E-6,
-0.105489265014994));
#38849=CARTESIAN_POINT('Ctrl Pts',(-0.121690006423613,-0.000494787113293386,
-0.105460485772185));
#38850=CARTESIAN_POINT('Ctrl Pts',(-0.121687340224093,-0.000980883949462602,
-0.105431706529376));
#38851=CARTESIAN_POINT('Ctrl Pts',(-0.121681480491707,-0.00146694228632414,
-0.105402927286567));
#38852=CARTESIAN_POINT('Ctrl Pts',(-0.121201495045295,-0.0412812055376695,
-0.103045546983664));
#38853=CARTESIAN_POINT('Ctrl Pts',(-0.0992939868802457,-0.0808371514881188,
-0.100688166680762));
#38854=CARTESIAN_POINT('Ctrl Pts',(-0.0657995057974866,-0.102366791614373,
-0.0983307863778601));
#38855=CARTESIAN_POINT('Ctrl Pts',(-0.0323050247147275,-0.123896431740628,
-0.0959734060749579));
#38856=CARTESIAN_POINT('Ctrl Pts',(0.0127764292857409,-0.127399766042687,
-0.0936160257720558));
#38857=CARTESIAN_POINT('Ctrl Pts',(0.0491949030024557,-0.111303165164919,
-0.0912586454691537));
#38858=CARTESIAN_POINT('Ctrl Pts',(0.0856133767191708,-0.0952065642871499,
-0.0889012651662515));
#38859=CARTESIAN_POINT('Ctrl Pts',(0.113368870152132,-0.0595100282295526,
-0.0865438848633493));
#38860=CARTESIAN_POINT('Ctrl Pts',(0.119993991851324,-0.0202479052800325,
-0.0841865045604471));
#38861=CARTESIAN_POINT('Ctrl Pts',(0.126619113550515,0.0190142176694876,
-0.081829124257545));
#38862=CARTESIAN_POINT('Ctrl Pts',(0.112113863515937,0.0618419275109303,
-0.0794717439546429));
#38863=CARTESIAN_POINT('Ctrl Pts',(0.0829938194035347,0.0889975450679775,
-0.0771143636517407));
#38864=CARTESIAN_POINT('Ctrl Pts',(0.0538737752911323,0.116153162625025,
-0.0747569833488385));
#38865=CARTESIAN_POINT('Ctrl Pts',(0.0101389371009058,0.127636687897676,
-0.0723996030459363));
#38866=CARTESIAN_POINT('Ctrl Pts',(-0.0285656586709824,0.118290015279103,
-0.0700422227430341));
#38867=CARTESIAN_POINT('Ctrl Pts',(-0.0672702544428707,0.10894334266053,
-0.0676848424401319));
#38868=CARTESIAN_POINT('Ctrl Pts',(-0.100944607796421,0.0787664721507315,
-0.0653274621372298));
#38869=CARTESIAN_POINT('Ctrl Pts',(-0.114462590277186,0.0413141787233953,
-0.0629700818343277));
#38870=CARTESIAN_POINT('Ctrl Pts',(-0.119204526097562,0.0281763919263629,
-0.0621431428945498));
#38871=CARTESIAN_POINT('Ctrl Pts',(-0.121466186405048,0.0141433520392691,
-0.0613162039547719));
#38872=CARTESIAN_POINT('Ctrl Pts',(-0.121376290077639,8.23099624828544E-5,
-0.060489265014994));
#38873=CARTESIAN_POINT('Origin',(0.,0.,-0.19));
#38874=CARTESIAN_POINT('',(-0.12142737051279,-0.000153818344799855,-0.00901073498500596));
#38875=CARTESIAN_POINT('',(-0.121436917850398,-0.000108937277296349,-0.015489265014994));
#38876=CARTESIAN_POINT('',(-0.1215,-1.48794586096403E-17,-0.19));
#38877=CARTESIAN_POINT('Ctrl Pts',(-0.12142737051279,-0.000153818344799855,
-0.00901073498500596));
#38878=CARTESIAN_POINT('Ctrl Pts',(-0.121186248580763,0.0289004463450801,
-0.010721917262475));
#38879=CARTESIAN_POINT('Ctrl Pts',(-0.110736371434051,0.058159765361451,
-0.012433099539944));
#38880=CARTESIAN_POINT('Ctrl Pts',(-0.0917563917866803,0.0799663543477724,
-0.014144281817413));
#38881=CARTESIAN_POINT('Ctrl Pts',(-0.0656089551521823,0.110007819846043,
-0.0165016621203151));
#38882=CARTESIAN_POINT('Ctrl Pts',(-0.023272481971744,0.12590496306751,
-0.0188590424232173));
#38883=CARTESIAN_POINT('Ctrl Pts',(0.0161960346634556,0.120596967837864,
-0.0212164227261194));
#38884=CARTESIAN_POINT('Ctrl Pts',(0.0556645512986556,0.115288972608218,
-0.0235738030290216));
#38885=CARTESIAN_POINT('Ctrl Pts',(0.092265111388617,0.0887758389274579,
-0.0259311833319238));
#38886=CARTESIAN_POINT('Ctrl Pts',(0.109577856214941,0.0529262964459767,
-0.028288563634826));
#38887=CARTESIAN_POINT('Ctrl Pts',(0.126890601041264,0.0170767539644958,
-0.0306459439377282));
#38888=CARTESIAN_POINT('Ctrl Pts',(0.124915530603951,-0.0281091973177056,
-0.0330033242406303));
#38889=CARTESIAN_POINT('Ctrl Pts',(0.104529032480174,-0.0623134685653849,
-0.0353607045435324));
#38890=CARTESIAN_POINT('Ctrl Pts',(0.0841425343563973,-0.0965177398130642,
-0.0377180848464346));
#38891=CARTESIAN_POINT('Ctrl Pts',(0.0453446085461563,-0.119740331026221,
-0.0400754651493368));
#38892=CARTESIAN_POINT('Ctrl Pts',(0.00556841104745733,-0.121561109575771,
-0.0424328454522389));
#38893=CARTESIAN_POINT('Ctrl Pts',(-0.0342077864512416,-0.12338188812532,
-0.0447902257551411));
#38894=CARTESIAN_POINT('Ctrl Pts',(-0.0749622556383988,-0.103800854011263,
-0.0471476060580432));
#38895=CARTESIAN_POINT('Ctrl Pts',(-0.0983916412117136,-0.0716076791421647,
-0.0495049863609454));
#38896=CARTESIAN_POINT('Ctrl Pts',(-0.113318793140995,-0.0510970084353631,
-0.0510069025689656));
#38897=CARTESIAN_POINT('Ctrl Pts',(-0.121213482223646,-0.0254669158975791,
-0.0525088187769857));
#38898=CARTESIAN_POINT('Ctrl Pts',(-0.121366197770921,7.70029837308187E-5,
-0.0540107349850059));
#38899=CARTESIAN_POINT('Ctrl Pts',(-0.121376290077639,8.23099624828544E-5,
-0.060489265014994));
#38900=CARTESIAN_POINT('Ctrl Pts',(-0.121209916175962,-0.0259408936475976,
-0.0589588236518697));
#38901=CARTESIAN_POINT('Ctrl Pts',(-0.112988979946086,-0.0520600104833506,
-0.0574283822887454));
#38902=CARTESIAN_POINT('Ctrl Pts',(-0.0975294472722496,-0.0727774231105138,
-0.0558979409256212));
#38903=CARTESIAN_POINT('Ctrl Pts',(-0.0737167101785676,-0.104689015172212,
-0.053540560622719));
#38904=CARTESIAN_POINT('Ctrl Pts',(-0.0327296243832231,-0.123784482950735,
-0.0511831803198168));
#38905=CARTESIAN_POINT('Ctrl Pts',(0.00702127041893494,-0.121487324712238,
-0.0488258000169147));
#38906=CARTESIAN_POINT('Ctrl Pts',(0.046772165221093,-0.119190166473741,
-0.0464684197140125));
#38907=CARTESIAN_POINT('Ctrl Pts',(0.0852868690300645,-0.0955003822182252,
-0.0441110394111104));
#38908=CARTESIAN_POINT('Ctrl Pts',(0.105264570463262,-0.0610573524762343,
-0.0417536591082082));
#38909=CARTESIAN_POINT('Ctrl Pts',(0.12524227189646,-0.0266143227342432,
-0.039396278805306));
#38910=CARTESIAN_POINT('Ctrl Pts',(0.126682970953884,0.0185819524942231,
-0.0370388985024038));
#38911=CARTESIAN_POINT('Ctrl Pts',(0.10894056031447,0.0542266326955117,
-0.0346815181995016));
#38912=CARTESIAN_POINT('Ctrl Pts',(0.0911981496750572,0.0898713128967998,
-0.0323241378965995));
#38913=CARTESIAN_POINT('Ctrl Pts',(0.0542726293388079,0.115964398070911,
-0.0299667575936974));
#38914=CARTESIAN_POINT('Ctrl Pts',(0.0147484614780834,0.120791518932237,
-0.0276093772907952));
#38915=CARTESIAN_POINT('Ctrl Pts',(-0.0247757063826414,0.125618639793563,
-0.0252519969878931));
#38916=CARTESIAN_POINT('Ctrl Pts',(-0.0668985217678414,0.109179796342103,
-0.0228946166849909));
#38917=CARTESIAN_POINT('Ctrl Pts',(-0.0926952692470915,0.078847151123733,
-0.0205372363820887));
#38918=CARTESIAN_POINT('Ctrl Pts',(-0.111108539616056,0.0571962357181767,
-0.0188545792597238));
#38919=CARTESIAN_POINT('Ctrl Pts',(-0.121203912684722,0.0284666277043547,
-0.0171719221373589));
#38920=CARTESIAN_POINT('Ctrl Pts',(-0.121436917850398,-0.000108937277296349,
-0.015489265014994));
#38921=CARTESIAN_POINT('Origin',(0.,0.,-0.466687266823562));
#38922=CARTESIAN_POINT('',(-0.0957194724394942,6.07309540377199E-5,-0.0391872668235621));
#38923=CARTESIAN_POINT('',(-0.095775248172958,-8.59169925714678E-5,-0.0303127331764374));
#38924=CARTESIAN_POINT('',(-0.095825,-3.71055914695333E-15,-0.466687266823562));
#38925=CARTESIAN_POINT('',(-0.0660853196898438,0.0695807828091147,-2.60208521396521E-17));
#38926=CARTESIAN_POINT('Ctrl Pts',(-0.0957194724394942,6.07309540377222E-5,
-0.0391872668235621));
#38927=CARTESIAN_POINT('Ctrl Pts',(-0.0955990282640391,-0.0200853268797188,
-0.037685350615542));
#38928=CARTESIAN_POINT('Ctrl Pts',(-0.079599763565718,-0.072026908170814,
-0.0338260541046197));
#38929=CARTESIAN_POINT('Ctrl Pts',(0.00516325821538433,-0.112752444638587,
-0.0276093772907953));
#38930=CARTESIAN_POINT('Ctrl Pts',(0.0969610666293677,-0.0578066470336301,
-0.0205372363820888));
#38931=CARTESIAN_POINT('Ctrl Pts',(0.101634180818392,0.0491055451050618,
-0.0134650954733823));
#38932=CARTESIAN_POINT('Ctrl Pts',(0.0178076722256624,0.109828753243069,
-0.00661935001268602));
#38933=CARTESIAN_POINT('Ctrl Pts',(-0.0453521829837652,0.0890152473756348,
-0.00213098485489195));
#38934=CARTESIAN_POINT('Ctrl Pts',(-0.0660853196898438,0.0695807828091147,
-3.4477629085039E-17));
#38935=CARTESIAN_POINT('',(0.0442442935173268,0.0849992536211503,0.));
#38936=CARTESIAN_POINT('Origin',(0.,0.,0.));
#38937=CARTESIAN_POINT('Ctrl Pts',(-0.095775248172958,-8.59169925714618E-5,
-0.0303127331764374));
#38938=CARTESIAN_POINT('Ctrl Pts',(-0.0958489363990951,-0.00912298142099969,
-0.0296380099959002));
#38939=CARTESIAN_POINT('Ctrl Pts',(-0.0905597458604163,-0.0496463906961603,
-0.0266059065124609));
#38940=CARTESIAN_POINT('Ctrl Pts',(-0.0334457163768884,-0.107772616556743,
-0.0212164227261194));
#38941=CARTESIAN_POINT('Ctrl Pts',(0.0715887019827832,-0.0873619805387618,
-0.014144281817413));
#38942=CARTESIAN_POINT('Ctrl Pts',(0.112228173818235,0.0118018015396153,
-0.00707214090870642));
#38943=CARTESIAN_POINT('Ctrl Pts',(0.0722220004899157,0.0704361389289412,
-0.00235738030290216));
#38944=CARTESIAN_POINT('Ctrl Pts',(0.0442442935173268,0.0849992536211503,
0.));
#38945=CARTESIAN_POINT('Origin',(0.,0.,-0.466687266823562));
#38946=CARTESIAN_POINT('',(-0.0959751130414699,-5.26327519415071E-8,-0.0841872668235621));
#38947=CARTESIAN_POINT('',(-0.0957274320715207,6.49164786371351E-5,-0.0753127331764374));
#38948=CARTESIAN_POINT('',(-0.095825,-3.71055914695333E-15,-0.466687266823562));
#38949=CARTESIAN_POINT('Ctrl Pts',(-0.09597511304147,-5.26327519511634E-8,
-0.0841872668235621));
#38950=CARTESIAN_POINT('Ctrl Pts',(-0.0959751130735191,-3.43738508333871E-6,
-0.0841870127358571));
#38951=CARTESIAN_POINT('Ctrl Pts',(-0.0959735887129596,-0.0314099491378808,
-0.08182937834525));
#38952=CARTESIAN_POINT('Ctrl Pts',(-0.0621635455577987,-0.0942160343945172,
-0.0771143636517407));
#38953=CARTESIAN_POINT('Ctrl Pts',(0.0443946751765518,-0.103778829919784,
-0.0700422227430341));
#38954=CARTESIAN_POINT('Ctrl Pts',(0.111070156606965,-0.0201100099317029,
-0.0629700818343277));
#38955=CARTESIAN_POINT('Ctrl Pts',(0.077962939724412,0.0816258135429839,
-0.0558979409256211));
#38956=CARTESIAN_POINT('Ctrl Pts',(-0.0251832945736545,0.110029895006483,
-0.0488258000169148));
#38957=CARTESIAN_POINT('Ctrl Pts',(-0.0886060442232168,0.0545484618118582,
-0.0432555753162283));
#38958=CARTESIAN_POINT('Ctrl Pts',(-0.0957880752463548,0.0115355582700803,
-0.0400427309184441));
#38959=CARTESIAN_POINT('Ctrl Pts',(-0.0957194724394942,6.07309540377222E-5,
-0.0391872668235621));
#38960=CARTESIAN_POINT('Ctrl Pts',(-0.0957274320715207,6.49164786371299E-5,
-0.0753127331764374));
#38961=CARTESIAN_POINT('Ctrl Pts',(-0.0955962157823984,-0.0204591451340034,
-0.0737822918133132));
#38962=CARTESIAN_POINT('Ctrl Pts',(-0.0791254621839689,-0.07278913840738,
-0.0698944701472868));
#38963=CARTESIAN_POINT('Ctrl Pts',(0.00651252049231818,-0.112687006408486,
-0.0636492681783584));
#38964=CARTESIAN_POINT('Ctrl Pts',(0.0976402116650261,-0.0566358069940454,
-0.0565771272696518));
#38965=CARTESIAN_POINT('Ctrl Pts',(0.101048976780522,0.0503008121113309,
-0.0495049863609453));
#38966=CARTESIAN_POINT('Ctrl Pts',(0.0136813721824698,0.112038340180693,
-0.0424328454522389));
#38967=CARTESIAN_POINT('Ctrl Pts',(-0.0764747035464821,0.076854043937596,
-0.0360354277240695));
#38968=CARTESIAN_POINT('Ctrl Pts',(-0.0955914809301527,0.0224511489692956,
-0.0319953902988024));
#38969=CARTESIAN_POINT('Ctrl Pts',(-0.095775248172958,-8.59169925714618E-5,
-0.0303127331764374));
#38970=CARTESIAN_POINT('Origin',(0.,0.,-0.466687266823562));
#38971=CARTESIAN_POINT('',(-0.0957194655585664,-6.0908243783317E-5,-0.129187266823562));
#38972=CARTESIAN_POINT('',(-0.0959744524639226,-6.84934123261483E-6,-0.120312733176437));
#38973=CARTESIAN_POINT('',(-0.095825,-3.71055914695333E-15,-0.466687266823562));
#38974=CARTESIAN_POINT('Ctrl Pts',(-0.0957194655585664,-6.09082437833235E-5,
-0.129187266823562));
#38975=CARTESIAN_POINT('Ctrl Pts',(-0.0957878927736574,-0.0115423430508919,
-0.12833129455327));
#38976=CARTESIAN_POINT('Ctrl Pts',(-0.0885997276627033,-0.0545612978206964,
-0.125117941980076));
#38977=CARTESIAN_POINT('Ctrl Pts',(-0.0251602537774947,-0.11003600414835,
-0.11954720910398));
#38978=CARTESIAN_POINT('Ctrl Pts',(0.0779805128909062,-0.081608819302419,
-0.112475068195273));
#38979=CARTESIAN_POINT('Ctrl Pts',(0.111065769910699,0.0201334402733364,
-0.105402927286567));
#38980=CARTESIAN_POINT('Ctrl Pts',(0.0443726347616168,0.10378839523891,
-0.0983307863778601));
#38981=CARTESIAN_POINT('Ctrl Pts',(-0.0621797921696317,0.0942030708531262,
-0.0912588995568586));
#38982=CARTESIAN_POINT('Ctrl Pts',(-0.0959748157271878,0.0313996896429778,
-0.0865443930387592));
#38983=CARTESIAN_POINT('Ctrl Pts',(-0.09597511304147,-5.26327519511634E-8,
-0.0841872668235621));
#38984=CARTESIAN_POINT('Ctrl Pts',(-0.0959744524639226,-6.84934123261998E-6,
-0.120312733176437));
#38985=CARTESIAN_POINT('Ctrl Pts',(-0.0959748548604342,-0.00039023024799691,
-0.120283953933628));
#38986=CARTESIAN_POINT('Ctrl Pts',(-0.0958005075262998,-0.0321769314557355,
-0.117897794387917));
#38987=CARTESIAN_POINT('Ctrl Pts',(-0.0610334100648855,-0.094952004625933,
-0.113154254539304));
#38988=CARTESIAN_POINT('Ctrl Pts',(0.0456315363448654,-0.103241066588768,
-0.106082113630597));
#38989=CARTESIAN_POINT('Ctrl Pts',(0.111302404448902,-0.0187812994845884,
-0.0990099727218907));
#38990=CARTESIAN_POINT('Ctrl Pts',(0.0769822665584455,0.082551176948899,
-0.0919378318131844));
#38991=CARTESIAN_POINT('Ctrl Pts',(-0.0264965203447265,0.109721764831659,
-0.0848656909044777));
#38992=CARTESIAN_POINT('Ctrl Pts',(-0.0889296549406001,0.053773055187859,
-0.0793239913588955));
#38993=CARTESIAN_POINT('Ctrl Pts',(-0.0957983317881795,0.0111546231206798,
-0.0761396721162153));
#38994=CARTESIAN_POINT('Ctrl Pts',(-0.0957274320715207,6.49164786371299E-5,
-0.0753127331764374));
#38995=CARTESIAN_POINT('Origin',(0.,0.,-0.466687266823562));
#38996=CARTESIAN_POINT('',(-0.0957878027106809,8.13637278885715E-5,-0.174187266823562));
#38997=CARTESIAN_POINT('',(-0.0957121716339357,-5.66137451362067E-5,-0.165312733176438));
#38998=CARTESIAN_POINT('',(-0.095825,-3.71055914695333E-15,-0.466687266823562));
#38999=CARTESIAN_POINT('Ctrl Pts',(-0.0957878027106809,8.13637278885707E-5,
-0.174187266823562));
#39000=CARTESIAN_POINT('Ctrl Pts',(-0.0955951522778602,-0.0228366251828878,
-0.172475576370683));
#39001=CARTESIAN_POINT('Ctrl Pts',(-0.0759427696888102,-0.077614637258398,
-0.168406505614902));
#39002=CARTESIAN_POINT('Ctrl Pts',(0.0150412165657262,-0.111869218970413,
-0.161980054556218));
#39003=CARTESIAN_POINT('Ctrl Pts',(0.101654099403055,-0.0490653075613788,
-0.154907913647512));
#39004=CARTESIAN_POINT('Ctrl Pts',(0.09694377988408,0.0578175049768839,
-0.147835772738805));
#39005=CARTESIAN_POINT('Ctrl Pts',(0.00514187719049035,0.112758686937953,
-0.140763631830099));
#39006=CARTESIAN_POINT('Ctrl Pts',(-0.0796090601597848,0.0720115357319004,
-0.134547463191685));
#39007=CARTESIAN_POINT('Ctrl Pts',(-0.0955994416115853,0.0200779666281811,
-0.130688674856172));
#39008=CARTESIAN_POINT('Ctrl Pts',(-0.0957194655585664,-6.09082437833235E-5,
-0.129187266823562));
#39009=CARTESIAN_POINT('Ctrl Pts',(-0.0957121716339357,-5.66137451362076E-5,
-0.165312733176438));
#39010=CARTESIAN_POINT('Ctrl Pts',(-0.0957775679602116,-0.0119229404138125,
-0.164428235751041));
#39011=CARTESIAN_POINT('Ctrl Pts',(-0.0882696983379308,-0.0553358580165303,
-0.161186358022743));
#39012=CARTESIAN_POINT('Ctrl Pts',(-0.0238437133266645,-0.110328764767113,
-0.155587099991542));
#39013=CARTESIAN_POINT('Ctrl Pts',(0.0789500302236065,-0.0806712564157815,
-0.148514959082836));
#39014=CARTESIAN_POINT('Ctrl Pts',(0.110817273075402,0.0214590532670084,
-0.14144281817413));
#39015=CARTESIAN_POINT('Ctrl Pts',(0.0431293735332865,0.104311151550646,
-0.134370677265423));
#39016=CARTESIAN_POINT('Ctrl Pts',(-0.0628716275040662,0.0934972072317672,
-0.127327315599526));
#39017=CARTESIAN_POINT('Ctrl Pts',(-0.0959418935481174,0.0310134659545147,
-0.122641334236531));
#39018=CARTESIAN_POINT('Ctrl Pts',(-0.0959744524639226,-6.84934123261998E-6,
-0.120312733176437));
#39019=CARTESIAN_POINT('Origin',(0.,0.,-0.466687266823562));
#39020=CARTESIAN_POINT('',(-0.095944975615187,-4.66871613868081E-5,-0.219187266823562));
#39021=CARTESIAN_POINT('',(-0.0957985183985989,8.23860933714532E-5,-0.210312733176438));
#39022=CARTESIAN_POINT('',(-0.095825,-3.71055914695333E-15,-0.466687266823562));
#39023=CARTESIAN_POINT('Ctrl Pts',(-0.095944975615187,-4.66871613868159E-5,
-0.219187266823562));
#39024=CARTESIAN_POINT('Ctrl Pts',(-0.0959619481171234,-0.00284686035185996,
-0.218977238490998));
#39025=CARTESIAN_POINT('Ctrl Pts',(-0.0945905159566559,-0.037059626206742,
-0.216409829855532));
#39026=CARTESIAN_POINT('Ctrl Pts',(-0.0536556310458891,-0.0993077717118213,
-0.211485040917164));
#39027=CARTESIAN_POINT('Ctrl Pts',(0.0533307801909408,-0.0994826028270216,
-0.204412900008458));
#39028=CARTESIAN_POINT('Ctrl Pts',(0.112406308710366,-0.0102850426384537,
-0.197340759099751));
#39029=CARTESIAN_POINT('Ctrl Pts',(0.0704991503786541,0.0881523120934825,
-0.190268618191045));
#39030=CARTESIAN_POINT('Ctrl Pts',(-0.0347424747368677,0.107396093029428,
-0.183196477282338));
#39031=CARTESIAN_POINT('Ctrl Pts',(-0.0908547496053409,0.0488523265191771,
-0.177836026826511));
#39032=CARTESIAN_POINT('Ctrl Pts',(-0.0958604749797034,0.00872656753663759,
-0.174832956673585));
#39033=CARTESIAN_POINT('Ctrl Pts',(-0.0957878027106809,8.13637278885707E-5,
-0.174187266823562));
#39034=CARTESIAN_POINT('Ctrl Pts',(-0.0957985183985989,8.23860933714523E-5,
-0.210312733176438));
#39035=CARTESIAN_POINT('Ctrl Pts',(-0.0955983110355252,-0.0232108787151331,
-0.208572517568454));
#39036=CARTESIAN_POINT('Ctrl Pts',(-0.0754156206185855,-0.078369269952436,
-0.204474921657569));
#39037=CARTESIAN_POINT('Ctrl Pts',(0.0163767894818392,-0.111681510260943,
-0.198019945443782));
#39038=CARTESIAN_POINT('Ctrl Pts',(0.102233084705024,-0.0478472083859376,
-0.190947804535075));
#39039=CARTESIAN_POINT('Ctrl Pts',(0.0962460332646973,0.058971688456773,
-0.183875663626369));
#39040=CARTESIAN_POINT('Ctrl Pts',(0.0037942348732942,0.112812068280055,
-0.176803522717662));
#39041=CARTESIAN_POINT('Ctrl Pts',(-0.0800771402773893,0.0712468149779357,
-0.170615879234352));
#39042=CARTESIAN_POINT('Ctrl Pts',(-0.0956032723579649,0.0197034317534234,
-0.166785616053944));
#39043=CARTESIAN_POINT('Ctrl Pts',(-0.0957121716339357,-5.66137451362076E-5,
-0.165312733176438));
#39044=CARTESIAN_POINT('Origin',(0.,0.,-0.466687266823562));
#39045=CARTESIAN_POINT('',(-0.0956804223565074,-2.35157469208761E-5,-0.264187266823562));
#39046=CARTESIAN_POINT('',(-0.0959371457461587,-5.20048528196981E-5,-0.255312733176438));
#39047=CARTESIAN_POINT('',(-0.095825,-3.71055914695333E-15,-0.466687266823562));
#39048=CARTESIAN_POINT('Ctrl Pts',(-0.0956804223565074,-2.35157469208793E-5,
-0.264187266823562));
#39049=CARTESIAN_POINT('Ctrl Pts',(-0.0957125021369695,-0.0143333873827806,
-0.263121520308411));
#39050=CARTESIAN_POINT('Ctrl Pts',(-0.0860327810025941,-0.0602547865702146,
-0.259698393490358));
#39051=CARTESIAN_POINT('Ctrl Pts',(-0.0154067542351519,-0.111819444898135,
-0.253917886369403));
#39052=CARTESIAN_POINT('Ctrl Pts',(0.0848414033458655,-0.0744506412347145,
-0.246845745460696));
#39053=CARTESIAN_POINT('Ctrl Pts',(0.108870415651418,0.0298025713485215,
-0.23977360455199));
#39054=CARTESIAN_POINT('Ctrl Pts',(0.0350932882052845,0.107281969135566,
-0.232701463643283));
#39055=CARTESIAN_POINT('Ctrl Pts',(-0.0670833532499771,0.0889435362384874,
-0.225839351067141));
#39056=CARTESIAN_POINT('Ctrl Pts',(-0.0957714469534591,0.0285825808256805,
-0.221334618793901));
#39057=CARTESIAN_POINT('Ctrl Pts',(-0.095944975615187,-4.66871613868159E-5,
-0.219187266823562));
#39058=CARTESIAN_POINT('Ctrl Pts',(-0.0959371457461587,-5.20048528197068E-5,
-0.255312733176438));
#39059=CARTESIAN_POINT('Ctrl Pts',(-0.0959581715766043,-0.00323317110377817,
-0.25507417968877));
#39060=CARTESIAN_POINT('Ctrl Pts',(-0.0943823518025523,-0.0378294848809537,
-0.2524782458982));
#39061=CARTESIAN_POINT('Ctrl Pts',(-0.0524652380640034,-0.0999417689982206,
-0.247524931804727));
#39062=CARTESIAN_POINT('Ctrl Pts',(0.0545156184897837,-0.0988382847881933,
-0.240452790896021));
#39063=CARTESIAN_POINT('Ctrl Pts',(0.112521167612446,-0.00894124253760813,
-0.233380649987314));
#39064=CARTESIAN_POINT('Ctrl Pts',(0.0694408433772929,0.0889883596604602,
-0.226308509078608));
#39065=CARTESIAN_POINT('Ctrl Pts',(-0.0360231939491006,0.106973307408655,
-0.219236368169901));
#39066=CARTESIAN_POINT('Ctrl Pts',(-0.091137108833105,0.0480783572787451,
-0.213904442869178));
#39067=CARTESIAN_POINT('Ctrl Pts',(-0.0958695216211795,0.00834330537444174,
-0.210929897871357));
#39068=CARTESIAN_POINT('Ctrl Pts',(-0.0957985183985989,8.23860933714523E-5,
-0.210312733176438));
#39069=CARTESIAN_POINT('Origin',(0.,0.,-0.466687266823562));
#39070=CARTESIAN_POINT('',(-0.0958690039724624,7.88897705069557E-5,-0.309187266823562));
#39071=CARTESIAN_POINT('',(-0.0956779014015301,-1.7615076390011E-5,-0.300312733176438));
#39072=CARTESIAN_POINT('',(-0.095825,-3.71055914695333E-15,-0.466687266823562));
#39073=CARTESIAN_POINT('Ctrl Pts',(-0.0958690039724624,7.88897705069598E-5,
-0.309187266823562));
#39074=CARTESIAN_POINT('Ctrl Pts',(-0.0956435931287137,-0.0255918778922679,
-0.307265802125824));
#39075=CARTESIAN_POINT('Ctrl Pts',(-0.0718951791629235,-0.0831279477414135,
-0.302986957125184));
#39076=CARTESIAN_POINT('Ctrl Pts',(0.0248005137658673,-0.110116804519884,
-0.296350731821642));
#39077=CARTESIAN_POINT('Ctrl Pts',(0.105567722156006,-0.0399555934234326,
-0.289278590912935));
#39078=CARTESIAN_POINT('Ctrl Pts',(0.0914958773173812,0.0661021680587838,
-0.282206450004229));
#39079=CARTESIAN_POINT('Ctrl Pts',(-0.00477332737082577,0.112774766988728,
-0.275134309095522));
#39080=CARTESIAN_POINT('Ctrl Pts',(-0.0828930919733463,0.0663682535192907,
-0.269127914701967));
#39081=CARTESIAN_POINT('Ctrl Pts',(-0.0956415431973834,0.0173193640471915,
-0.265478900611313));
#39082=CARTESIAN_POINT('Ctrl Pts',(-0.0956804223565074,-2.35157469208793E-5,
-0.264187266823562));
#39083=CARTESIAN_POINT('Ctrl Pts',(-0.09567790140153,-1.76150763900179E-5,
-0.300312733176438));
#39084=CARTESIAN_POINT('Ctrl Pts',(-0.0957026375134359,-0.0147114989746946,
-0.299218461506183));
#39085=CARTESIAN_POINT('Ctrl Pts',(-0.0856582592510746,-0.0610282955341015,
-0.295766809533026));
#39086=CARTESIAN_POINT('Ctrl Pts',(-0.0140695777255182,-0.111995438526656,
-0.289957777256965));
#39087=CARTESIAN_POINT('Ctrl Pts',(0.0857248891793926,-0.0734316658894842,
-0.28288563634826));
#39088=CARTESIAN_POINT('Ctrl Pts',(0.108506554426889,0.0311012876396027,
-0.275813495439553));
#39089=CARTESIAN_POINT('Ctrl Pts',(0.0338089402553138,0.107693595438131,
-0.268741354530847));
#39090=CARTESIAN_POINT('Ctrl Pts',(-0.0677174862885282,0.0882169577300349,
-0.261907767109808));
#39091=CARTESIAN_POINT('Ctrl Pts',(-0.0957503947839486,0.0282030436150841,
-0.257431559991672));
#39092=CARTESIAN_POINT('Ctrl Pts',(-0.0959371457461587,-5.20048528197068E-5,
-0.255312733176438));
#39093=CARTESIAN_POINT('Origin',(0.,0.,-0.466687266823562));
#39094=CARTESIAN_POINT('',(-0.0958726565381089,-8.61752489211661E-5,-0.354187266823562));
#39095=CARTESIAN_POINT('',(-0.0958786240325138,8.20367901696907E-5,-0.345312733176438));
#39096=CARTESIAN_POINT('',(-0.095825,-3.71055914695333E-15,-0.466687266823562));
#39097=CARTESIAN_POINT('Ctrl Pts',(-0.095872656538109,-8.6175248921171E-5,
-0.354187266823562));
#39098=CARTESIAN_POINT('Ctrl Pts',(-0.0959221857987575,-0.00567877154923316,
-0.353767464246139));
#39099=CARTESIAN_POINT('Ctrl Pts',(-0.0929422356532186,-0.0426364993896563,
-0.350990281365814));
#39100=CARTESIAN_POINT('Ctrl Pts',(-0.0447352950033125,-0.103710198939767,
-0.345855718182587));
#39101=CARTESIAN_POINT('Ctrl Pts',(0.0618562700166257,-0.0943788386242131,
-0.338783577273881));
#39102=CARTESIAN_POINT('Ctrl Pts',(0.112874708577635,-0.000401788756397879,
-0.331711436365174));
#39103=CARTESIAN_POINT('Ctrl Pts',(0.06249144654252,0.0940099781523149,
-0.324639295456468));
#39104=CARTESIAN_POINT('Ctrl Pts',(-0.0440333363121848,0.103927081651485,
-0.317567154547761));
#39105=CARTESIAN_POINT('Ctrl Pts',(-0.0928049870134241,0.0431662527422258,
-0.312416478336793));
#39106=CARTESIAN_POINT('Ctrl Pts',(-0.0959201420987464,0.00590272209691865,
-0.309623182428726));
#39107=CARTESIAN_POINT('Ctrl Pts',(-0.0958690039724624,7.88897705069598E-5,
-0.309187266823562));
#39108=CARTESIAN_POINT('Ctrl Pts',(-0.0958786240325138,8.20367901696933E-5,
-0.345312733176438));
#39109=CARTESIAN_POINT('Ctrl Pts',(-0.0956537848124931,-0.0259620098340212,
-0.343362743323596));
#39110=CARTESIAN_POINT('Ctrl Pts',(-0.07131568583194,-0.0838783814842911,
-0.339055373167851));
#39111=CARTESIAN_POINT('Ctrl Pts',(0.0261155403145056,-0.109807778273315,
-0.332390622709205));
#39112=CARTESIAN_POINT('Ctrl Pts',(0.106037008942776,-0.0386939290059783,
-0.325318481800498));
#39113=CARTESIAN_POINT('Ctrl Pts',(0.0906998339925985,0.0671920060838559,
-0.318246340891792));
#39114=CARTESIAN_POINT('Ctrl Pts',(-0.00612061239846709,0.112708972315148,
-0.311174199983085));
#39115=CARTESIAN_POINT('Ctrl Pts',(-0.0833117710540488,0.0655980927825272,
-0.305196330744634));
#39116=CARTESIAN_POINT('Ctrl Pts',(-0.0956493487145368,0.0169434121562133,
-0.301575841809085));
#39117=CARTESIAN_POINT('Ctrl Pts',(-0.09567790140153,-1.76150763900179E-5,
-0.300312733176438));
#39118=CARTESIAN_POINT('Ctrl Pts',(0.0534655244842089,-0.079522753452257,
-0.374823468161444));
#39119=CARTESIAN_POINT('Ctrl Pts',(0.0796406283699102,-0.0619244486033452,
-0.372466087858542));
#39120=CARTESIAN_POINT('Ctrl Pts',(0.112844070495072,0.00081318648518734,
-0.367751327252737));
#39121=CARTESIAN_POINT('Ctrl Pts',(0.0613779578258757,0.0948145779316648,
-0.360679186344031));
#39122=CARTESIAN_POINT('Ctrl Pts',(-0.0452794177261462,0.103360181665046,
-0.353607045435324));
#39123=CARTESIAN_POINT('Ctrl Pts',(-0.111232369054601,0.0191891251444319,
-0.346534904526618));
#39124=CARTESIAN_POINT('Ctrl Pts',(-0.0772712803160827,-0.0822934176220715,
-0.339462763617911));
#39125=CARTESIAN_POINT('Ctrl Pts',(0.0261155403145056,-0.109807778273315,
-0.332390622709205));
#39126=CARTESIAN_POINT('Ctrl Pts',(0.106037008942776,-0.0386939290059783,
-0.325318481800498));
#39127=CARTESIAN_POINT('Ctrl Pts',(0.0906998339925985,0.0671920060838559,
-0.318246340891792));
#39128=CARTESIAN_POINT('Ctrl Pts',(-0.00612061239846709,0.112708972315148,
-0.311174199983085));
#39129=CARTESIAN_POINT('Ctrl Pts',(-0.0974419058465003,0.0569742673395502,
-0.304102059074378));
#39130=CARTESIAN_POINT('Ctrl Pts',(-0.101224411638868,-0.0499460644092083,
-0.297029918165673));
#39131=CARTESIAN_POINT('Ctrl Pts',(-0.0140695777255182,-0.111995438526656,
-0.289957777256965));
#39132=CARTESIAN_POINT('Ctrl Pts',(0.0857248891793926,-0.0734316658894842,
-0.28288563634826));
#39133=CARTESIAN_POINT('Ctrl Pts',(0.108506554426889,0.0311012876396027,
-0.275813495439553));
#39134=CARTESIAN_POINT('Ctrl Pts',(0.0338089402553138,0.107693595438131,
-0.268741354530847));
#39135=CARTESIAN_POINT('Ctrl Pts',(-0.0712616691093911,0.0875370483988087,
-0.261669213622139));
#39136=CARTESIAN_POINT('Ctrl Pts',(-0.112312792499519,-0.0112603696058821,
-0.254597072713434));
#39137=CARTESIAN_POINT('Ctrl Pts',(-0.0524652380640034,-0.0999417689982206,
-0.247524931804727));
#39138=CARTESIAN_POINT('Ctrl Pts',(0.0545156184897837,-0.0988382847881933,
-0.240452790896021));
#39139=CARTESIAN_POINT('Ctrl Pts',(0.112521167612446,-0.00894124253760813,
-0.233380649987314));
#39140=CARTESIAN_POINT('Ctrl Pts',(0.0694408433772929,0.0889883596604602,
-0.226308509078608));
#39141=CARTESIAN_POINT('Ctrl Pts',(-0.0360231939491006,0.106973307408655,
-0.219236368169901));
#39142=CARTESIAN_POINT('Ctrl Pts',(-0.109125000539913,0.0288564241744764,
-0.212164227261195));
#39143=CARTESIAN_POINT('Ctrl Pts',(-0.0841919557899689,-0.0751842638507629,
-0.205092086352488));
#39144=CARTESIAN_POINT('Ctrl Pts',(0.0163767894818392,-0.111681510260943,
-0.198019945443782));
#39145=CARTESIAN_POINT('Ctrl Pts',(0.102233084705024,-0.0478472083859376,
-0.190947804535075));
#39146=CARTESIAN_POINT('Ctrl Pts',(0.0962460332646973,0.058971688456773,
-0.183875663626369));
#39147=CARTESIAN_POINT('Ctrl Pts',(0.0037942348732942,0.112812068280055,
-0.176803522717662));
#39148=CARTESIAN_POINT('Ctrl Pts',(-0.0920661980803001,0.0653052380866966,
-0.169731381808956));
#39149=CARTESIAN_POINT('Ctrl Pts',(-0.105216931285724,-0.0408699930240835,
-0.162659240900249));
#39150=CARTESIAN_POINT('Ctrl Pts',(-0.0238437133266645,-0.110328764767113,
-0.155587099991542));
#39151=CARTESIAN_POINT('Ctrl Pts',(0.0789500302236065,-0.0806712564157815,
-0.148514959082836));
#39152=CARTESIAN_POINT('Ctrl Pts',(0.110817273075402,0.0214590532670084,
-0.14144281817413));
#39153=CARTESIAN_POINT('Ctrl Pts',(0.0431293735332865,0.104311151550646,
-0.134370677265423));
#39154=CARTESIAN_POINT('Ctrl Pts',(-0.0633047486032753,0.0934530213523478,
-0.127298536356717));
#39155=CARTESIAN_POINT('Ctrl Pts',(-0.112867656235649,-0.00136068312712246,
-0.12022639544801));
#39156=CARTESIAN_POINT('Ctrl Pts',(-0.0610334100648855,-0.094952004625933,
-0.113154254539304));
#39157=CARTESIAN_POINT('Ctrl Pts',(0.0456315363448654,-0.103241066588768,
-0.106082113630597));
#39158=CARTESIAN_POINT('Ctrl Pts',(0.111302404448902,-0.0187812994845884,
-0.0990099727218907));
#39159=CARTESIAN_POINT('Ctrl Pts',(0.0769822665584455,0.082551176948899,
-0.0919378318131844));
#39160=CARTESIAN_POINT('Ctrl Pts',(-0.0264965203447265,0.109721764831659,
-0.0848656909044777));
#39161=CARTESIAN_POINT('Ctrl Pts',(-0.106171703310255,0.038321798989649,
-0.0777935499957714));
#39162=CARTESIAN_POINT('Ctrl Pts',(-0.090464948553087,-0.0675061866584397,
-0.0707214090870648));
#39163=CARTESIAN_POINT('Ctrl Pts',(0.00651252049231818,-0.112687006408486,
-0.0636492681783584));
#39164=CARTESIAN_POINT('Ctrl Pts',(0.0976402116650261,-0.0566358069940454,
-0.0565771272696518));
#39165=CARTESIAN_POINT('Ctrl Pts',(0.101048976780522,0.0503008121113309,
-0.0495049863609453));
#39166=CARTESIAN_POINT('Ctrl Pts',(0.0136813721824698,0.112038340180693,
-0.0424328454522389));
#39167=CARTESIAN_POINT('Ctrl Pts',(-0.0859832891579445,0.0731432247798018,
-0.0353607045435324));
#39168=CARTESIAN_POINT('Ctrl Pts',(-0.108391384716252,-0.0314987328094481,
-0.0282885636348259));
#39169=CARTESIAN_POINT('Ctrl Pts',(-0.0334457163768884,-0.107772616556743,
-0.0212164227261194));
#39170=CARTESIAN_POINT('Ctrl Pts',(0.0715887019827832,-0.0873619805387618,
-0.014144281817413));
#39171=CARTESIAN_POINT('Ctrl Pts',(0.112228173818235,0.0118018015396153,
-0.00707214090870642));
#39172=CARTESIAN_POINT('Ctrl Pts',(0.0722220004899157,0.0704361389289412,
-0.00235738030290216));
#39173=CARTESIAN_POINT('Ctrl Pts',(0.0442442935173268,0.0849992536211503,
0.));
#39174=CARTESIAN_POINT('Ctrl Pts',(0.0582406435071917,-0.0866250986818831,
-0.369882312107629));
#39175=CARTESIAN_POINT('Ctrl Pts',(0.0867535012576304,-0.0674550520223937,
-0.367524931804727));
#39176=CARTESIAN_POINT('Ctrl Pts',(0.122922412994284,0.000885813889333945,
-0.362810171198922));
#39177=CARTESIAN_POINT('Ctrl Pts',(0.0668597529982539,0.103282668333945,
-0.355738030290216));
#39178=CARTESIAN_POINT('Ctrl Pts',(-0.0493234182483436,0.112591498002988,
-0.34866588938151));
#39179=CARTESIAN_POINT('Ctrl Pts',(-0.121166767090871,0.0209029464787511,
-0.341593748472803));
#39180=CARTESIAN_POINT('Ctrl Pts',(-0.0841725417200849,-0.0896432167261558,
-0.334521607564097));
#39181=CARTESIAN_POINT('Ctrl Pts',(0.0284479744307761,-0.119614943095186,
-0.32744946665539));
#39182=CARTESIAN_POINT('Ctrl Pts',(0.115507398383964,-0.0421497656082171,
-0.320377325746683));
#39183=CARTESIAN_POINT('Ctrl Pts',(0.0988004279147136,0.0731930661976151,
-0.313305184837978));
#39184=CARTESIAN_POINT('Ctrl Pts',(-0.00666725723134143,0.1227752489103,
-0.30623304392927));
#39185=CARTESIAN_POINT('Ctrl Pts',(-0.10614464845928,0.0620627596047666,
-0.299160903020565));
#39186=CARTESIAN_POINT('Ctrl Pts',(-0.110264977840549,-0.0544068530124132,
-0.292088762111858));
#39187=CARTESIAN_POINT('Ctrl Pts',(-0.0153261614566349,-0.121997987910679,
-0.285016621203151));
#39188=CARTESIAN_POINT('Ctrl Pts',(0.0933811602627245,-0.07999000321173,
-0.277944480294445));
#39189=CARTESIAN_POINT('Ctrl Pts',(0.118197504196123,0.0338790093898305,
-0.270872339385739));
#39190=CARTESIAN_POINT('Ctrl Pts',(0.0368284881848912,0.117311938121404,
-0.263800198477032));
#39191=CARTESIAN_POINT('Ctrl Pts',(-0.0776261994316225,0.0953551672531074,
-0.256728057568326));
#39192=CARTESIAN_POINT('Ctrl Pts',(-0.122343685437775,-0.0122660570208953,
-0.249655916659619));
#39193=CARTESIAN_POINT('Ctrl Pts',(-0.0571510193920957,-0.108867779674033,
-0.242583775750913));
#39194=CARTESIAN_POINT('Ctrl Pts',(0.0593845236284047,-0.107665740956336,
-0.235511634842206));
#39195=CARTESIAN_POINT('Ctrl Pts',(0.122570670972563,-0.00973980381129516,
-0.2284394939335));
#39196=CARTESIAN_POINT('Ctrl Pts',(0.0756427519039894,0.0969360981917489,
-0.221367353024793));
#39197=CARTESIAN_POINT('Ctrl Pts',(-0.0392405015572163,0.116527319645258,
-0.214295212116087));
#39198=CARTESIAN_POINT('Ctrl Pts',(-0.118871185038956,0.0314336524227755,
-0.20722307120738));
#39199=CARTESIAN_POINT('Ctrl Pts',(-0.0917113173515221,-0.0818991294020917,
-0.200150930298673));
#39200=CARTESIAN_POINT('Ctrl Pts',(0.0178394351725813,-0.12165602204788,
-0.193078789389967));
#39201=CARTESIAN_POINT('Ctrl Pts',(0.111363737630675,-0.05212054372052,
-0.186006648481261));
#39202=CARTESIAN_POINT('Ctrl Pts',(0.104841969969006,0.0642385746247095,
-0.178934507572554));
#39203=CARTESIAN_POINT('Ctrl Pts',(0.00413310601120864,0.122887552593788,
-0.171862366663848));
#39204=CARTESIAN_POINT('Ctrl Pts',(-0.100288824867713,0.0711377869618198,
-0.164790225755141));
#39205=CARTESIAN_POINT('Ctrl Pts',(-0.114614077857638,-0.0445201785041887,
-0.157718084846435));
#39206=CARTESIAN_POINT('Ctrl Pts',(-0.0259732457717892,-0.120182459994161,
-0.150645943937728));
#39207=CARTESIAN_POINT('Ctrl Pts',(0.0860012243308889,-0.0878761768731265,
-0.143573803029022));
#39208=CARTESIAN_POINT('Ctrl Pts',(0.120714598012218,0.0233756066808019,
-0.136501662120315));
#39209=CARTESIAN_POINT('Ctrl Pts',(0.0469813490632185,0.113627401019514,
-0.129429521211609));
#39210=CARTESIAN_POINT('Ctrl Pts',(-0.0689586295334048,0.101799508258067,
-0.122357380302902));
#39211=CARTESIAN_POINT('Ctrl Pts',(-0.122948105227214,-0.00148220861382132,
-0.115285239394196));
#39212=CARTESIAN_POINT('Ctrl Pts',(-0.0664844329483225,-0.103432368896811,
-0.108213098485489));
#39213=CARTESIAN_POINT('Ctrl Pts',(0.0497069853253135,-0.112461744507428,
-0.101140957576783));
#39214=CARTESIAN_POINT('Ctrl Pts',(0.121243057494299,-0.0204586970470439,
-0.0940688166680762));
#39215=CARTESIAN_POINT('Ctrl Pts',(0.0838577155327499,0.0899239970833903,
-0.0869966757593699));
#39216=CARTESIAN_POINT('Ctrl Pts',(-0.0288629805929245,0.119521247611216,
-0.0799245348506631));
#39217=CARTESIAN_POINT('Ctrl Pts',(-0.11565412259016,0.0417443998734104,
-0.0728523939419568));
#39218=CARTESIAN_POINT('Ctrl Pts',(-0.0985445643600286,-0.0735353069035231,
-0.0657802530332502));
#39219=CARTESIAN_POINT('Ctrl Pts',(0.00709416746558592,-0.122751321182076,
-0.0587081121245439));
#39220=CARTESIAN_POINT('Ctrl Pts',(0.106360665389696,-0.0616940706502668,
-0.0516359712158373));
#39221=CARTESIAN_POINT('Ctrl Pts',(0.110073874524117,0.0547932839817835,
-0.0445638303071308));
#39222=CARTESIAN_POINT('Ctrl Pts',(0.0149032844558327,0.122044721202136,
-0.0374916893984243));
#39223=CARTESIAN_POINT('Ctrl Pts',(-0.0936626384896434,0.0796758008167494,
-0.0304195484897179));
#39224=CARTESIAN_POINT('Ctrl Pts',(-0.118072048435149,-0.0343119512280323,
-0.0233474075810114));
#39225=CARTESIAN_POINT('Ctrl Pts',(-0.0364328240139933,-0.117398016783178,
-0.0162752666723049));
#39226=CARTESIAN_POINT('Ctrl Pts',(0.0779824403023166,-0.0951644637123691,
-0.00920312576359843));
#39227=CARTESIAN_POINT('Ctrl Pts',(0.122251509283174,0.0128558453852698,
-0.00213098485489189));
#39228=CARTESIAN_POINT('Ctrl Pts',(0.0786723000379761,0.0767269394055061,
0.00258377575091239));
#39229=CARTESIAN_POINT('Ctrl Pts',(0.0481958449080824,0.0925907166587118,
0.00494115605381455));
#39230=CARTESIAN_POINT('Ctrl Pts',(0.0630157625301746,-0.0937274439115092,
-0.364941156053815));
#39231=CARTESIAN_POINT('Ctrl Pts',(0.0938663741453508,-0.0729856554414422,
-0.362583775750912));
#39232=CARTESIAN_POINT('Ctrl Pts',(0.133000755493496,0.000958441293480677,
-0.357869015145108));
#39233=CARTESIAN_POINT('Ctrl Pts',(0.0723415481706322,0.111750758736225,
-0.350796874236402));
#39234=CARTESIAN_POINT('Ctrl Pts',(-0.053367418770541,0.121822814340931,
-0.343724733327695));
#39235=CARTESIAN_POINT('Ctrl Pts',(-0.131101165127142,0.0226167678130703,
-0.336652592418989));
#39236=CARTESIAN_POINT('Ctrl Pts',(-0.091073803124087,-0.09699301583024,
-0.329580451510282));
#39237=CARTESIAN_POINT('Ctrl Pts',(0.0307804085470464,-0.129422107917057,
-0.322508310601576));
#39238=CARTESIAN_POINT('Ctrl Pts',(0.124977787825153,-0.0456056022104559,
-0.315436169692869));
#39239=CARTESIAN_POINT('Ctrl Pts',(0.106901021836829,0.0791941263113741,
-0.308364028784163));
#39240=CARTESIAN_POINT('Ctrl Pts',(-0.00721390206421565,0.132841525505452,
-0.301291887875456));
#39241=CARTESIAN_POINT('Ctrl Pts',(-0.11484739107206,0.0671512518699828,
-0.29421974696675));
#39242=CARTESIAN_POINT('Ctrl Pts',(-0.119305544042229,-0.0588676416156181,
-0.287147606058043));
#39243=CARTESIAN_POINT('Ctrl Pts',(-0.0165827451877516,-0.132000537294701,
-0.280075465149337));
#39244=CARTESIAN_POINT('Ctrl Pts',(0.101037431346056,-0.0865483405339757,
-0.27300332424063));
#39245=CARTESIAN_POINT('Ctrl Pts',(0.127888453965356,0.0366567311400581,
-0.265931183331924));
#39246=CARTESIAN_POINT('Ctrl Pts',(0.0398480361144687,0.126930280804678,
-0.258859042423217));
#39247=CARTESIAN_POINT('Ctrl Pts',(-0.0839907297538541,0.103173286107406,
-0.251786901514511));
#39248=CARTESIAN_POINT('Ctrl Pts',(-0.132374578376031,-0.0132717444359084,
-0.244714760605805));
#39249=CARTESIAN_POINT('Ctrl Pts',(-0.0618368007201881,-0.117793790349846,
-0.237642619697098));
#39250=CARTESIAN_POINT('Ctrl Pts',(0.0642534287670256,-0.116493197124479,
-0.230570478788392));
#39251=CARTESIAN_POINT('Ctrl Pts',(0.13262017433268,-0.0105383650849823,
-0.223498337879685));
#39252=CARTESIAN_POINT('Ctrl Pts',(0.0818446604306858,0.104883836723038,
-0.216426196970978));
#39253=CARTESIAN_POINT('Ctrl Pts',(-0.0424578091653319,0.12608133188186,
-0.209354056062272));
#39254=CARTESIAN_POINT('Ctrl Pts',(-0.128617369537998,0.0340108806710746,
-0.202281915153565));
#39255=CARTESIAN_POINT('Ctrl Pts',(-0.0992306789130754,-0.0886139949534205,
-0.195209774244859));
#39256=CARTESIAN_POINT('Ctrl Pts',(0.0193020808633235,-0.131630533834817,
-0.188137633336152));
#39257=CARTESIAN_POINT('Ctrl Pts',(0.120494390556325,-0.0563938790551023,
-0.181065492427446));
#39258=CARTESIAN_POINT('Ctrl Pts',(0.113437906673315,0.0695054607926461,
-0.173993351518739));
#39259=CARTESIAN_POINT('Ctrl Pts',(0.00447197714912307,0.132963036907521,
-0.166921210610033));
#39260=CARTESIAN_POINT('Ctrl Pts',(-0.108511451655127,0.076970335836943,
-0.159849069701326));
#39261=CARTESIAN_POINT('Ctrl Pts',(-0.124011224429552,-0.048170363984294,
-0.15277692879262));
#39262=CARTESIAN_POINT('Ctrl Pts',(-0.0281027782169139,-0.130036155221209,
-0.145704787883913));
#39263=CARTESIAN_POINT('Ctrl Pts',(0.0930524184381714,-0.0950810973304716,
-0.138632646975207));
#39264=CARTESIAN_POINT('Ctrl Pts',(0.130611922949033,0.0252921600945957,
-0.1315605060665));
#39265=CARTESIAN_POINT('Ctrl Pts',(0.0508333245931506,0.122943650488382,
-0.124488365157794));
#39266=CARTESIAN_POINT('Ctrl Pts',(-0.0746125104635343,0.110145995163786,
-0.117416224249088));
#39267=CARTESIAN_POINT('Ctrl Pts',(-0.13302855421878,-0.00160373410052023,
-0.110344083340381));
#39268=CARTESIAN_POINT('Ctrl Pts',(-0.0719354558317593,-0.11191273316769,
-0.103271942431675));
#39269=CARTESIAN_POINT('Ctrl Pts',(0.0537824343057615,-0.121682422426087,
-0.0961998015229681));
#39270=CARTESIAN_POINT('Ctrl Pts',(0.131183710539696,-0.0221360946094997,
-0.0891276606142618));
#39271=CARTESIAN_POINT('Ctrl Pts',(0.0907331645070544,0.0972968172178819,
-0.0820555197055552));
#39272=CARTESIAN_POINT('Ctrl Pts',(-0.0312294408411226,0.129320730390771,
-0.0749833787968487));
#39273=CARTESIAN_POINT('Ctrl Pts',(-0.125136541870065,0.0451670007571721,
-0.0679112378881423));
#39274=CARTESIAN_POINT('Ctrl Pts',(-0.106624180166971,-0.0795644271486066,
-0.0608390969794357));
#39275=CARTESIAN_POINT('Ctrl Pts',(0.00767581443885381,-0.132815635955666,
-0.0537669560707293));
#39276=CARTESIAN_POINT('Ctrl Pts',(0.115081119114366,-0.066752334306488,
-0.0466948151620227));
#39277=CARTESIAN_POINT('Ctrl Pts',(0.119098772267712,0.0592857558522358,
-0.0396226742533163));
#39278=CARTESIAN_POINT('Ctrl Pts',(0.0161251967291956,0.132051102223579,
-0.0325505333446097));
#39279=CARTESIAN_POINT('Ctrl Pts',(-0.101341987821342,0.0862083768536969,
-0.0254783924359033));
#39280=CARTESIAN_POINT('Ctrl Pts',(-0.127752712154045,-0.0371251696466164,
-0.0184062515271968));
#39281=CARTESIAN_POINT('Ctrl Pts',(-0.0394199316510981,-0.127023417009613,
-0.0113341106184904));
#39282=CARTESIAN_POINT('Ctrl Pts',(0.0843761786218501,-0.102966946885977,
-0.00426196970978389));
#39283=CARTESIAN_POINT('Ctrl Pts',(0.132274844748113,0.0139098892309243,
0.00281017119892267));
#39284=CARTESIAN_POINT('Ctrl Pts',(0.0851225995860365,0.083017739882071,
0.00752493180472693));
#39285=CARTESIAN_POINT('Ctrl Pts',(0.0521473962988379,0.100182179696273,
0.00988231210762909));
#39286=CARTESIAN_POINT('Ctrl Pts',(0.0677908815531574,-0.100829789141135,
-0.36));
#39287=CARTESIAN_POINT('Ctrl Pts',(0.100979247033071,-0.0785162588604907,
-0.357642619697098));
#39288=CARTESIAN_POINT('Ctrl Pts',(0.143079097992708,0.00103106869762737,
-0.352927859091293));
#39289=CARTESIAN_POINT('Ctrl Pts',(0.0778233433430106,0.120218849138505,
-0.345855718182587));
#39290=CARTESIAN_POINT('Ctrl Pts',(-0.0574114192927385,0.131054130678874,
-0.338783577273881));
#39291=CARTESIAN_POINT('Ctrl Pts',(-0.141035563163412,0.0243305891473894,
-0.331711436365174));
#39292=CARTESIAN_POINT('Ctrl Pts',(-0.0979750645280892,-0.104342814934324,
-0.324639295456468));
#39293=CARTESIAN_POINT('Ctrl Pts',(0.0331128426633168,-0.139229272738928,
-0.317567154547761));
#39294=CARTESIAN_POINT('Ctrl Pts',(0.134448177266342,-0.0490614388126946,
-0.310495013639055));
#39295=CARTESIAN_POINT('Ctrl Pts',(0.115001615758944,0.0851951864251332,
-0.303422872730348));
#39296=CARTESIAN_POINT('Ctrl Pts',(-0.00776054689708998,0.142907802100605,
-0.296350731821642));
#39297=CARTESIAN_POINT('Ctrl Pts',(-0.123550133684839,0.072239744135199,
-0.289278590912935));
#39298=CARTESIAN_POINT('Ctrl Pts',(-0.128346110243909,-0.0633284302188229,
-0.282206450004229));
#39299=CARTESIAN_POINT('Ctrl Pts',(-0.0178393289188684,-0.142003086678724,
-0.275134309095522));
#39300=CARTESIAN_POINT('Ctrl Pts',(0.108693702429388,-0.0931066778562214,
-0.268062168186816));
#39301=CARTESIAN_POINT('Ctrl Pts',(0.13757940373459,0.0394344528902857,
-0.260990027278109));
#39302=CARTESIAN_POINT('Ctrl Pts',(0.0428675840440462,0.136548623487951,
-0.253917886369403));
#39303=CARTESIAN_POINT('Ctrl Pts',(-0.0903552600760858,0.110991404961705,
-0.246845745460696));
#39304=CARTESIAN_POINT('Ctrl Pts',(-0.142405471314287,-0.0142774318509216,
-0.23977360455199));
#39305=CARTESIAN_POINT('Ctrl Pts',(-0.0665225820482806,-0.126719801025659,
-0.232701463643283));
#39306=CARTESIAN_POINT('Ctrl Pts',(0.0691223339056467,-0.125320653292622,
-0.225629322734577));
#39307=CARTESIAN_POINT('Ctrl Pts',(0.142669677692796,-0.0113369263586695,
-0.21855718182587));
#39308=CARTESIAN_POINT('Ctrl Pts',(0.0880465689573824,0.112831575254327,
-0.211485040917164));
#39309=CARTESIAN_POINT('Ctrl Pts',(-0.0456751167734476,0.135635344118462,
-0.204412900008457));
#39310=CARTESIAN_POINT('Ctrl Pts',(-0.138363554037041,0.0365881089193739,
-0.197340759099751));
#39311=CARTESIAN_POINT('Ctrl Pts',(-0.106750040474629,-0.0953288605047495,
-0.190268618191044));
#39312=CARTESIAN_POINT('Ctrl Pts',(0.0207647265540655,-0.141605045621754,
-0.183196477282338));
#39313=CARTESIAN_POINT('Ctrl Pts',(0.129625043481976,-0.0606672143896846,
-0.176124336373631));
#39314=CARTESIAN_POINT('Ctrl Pts',(0.122033843377623,0.0747723469605826,
-0.169052195464925));
#39315=CARTESIAN_POINT('Ctrl Pts',(0.00481084828703748,0.143038521221254,
-0.161980054556218));
#39316=CARTESIAN_POINT('Ctrl Pts',(-0.11673407844254,0.0828028847120661,
-0.154907913647512));
#39317=CARTESIAN_POINT('Ctrl Pts',(-0.133408371001466,-0.0518205494643991,
-0.147835772738805));
#39318=CARTESIAN_POINT('Ctrl Pts',(-0.0302323106620386,-0.139889850448257,
-0.140763631830099));
#39319=CARTESIAN_POINT('Ctrl Pts',(0.100103612545454,-0.102286017787817,
-0.133691490921393));
#39320=CARTESIAN_POINT('Ctrl Pts',(0.140509247885848,0.0272087135083893,
-0.126619350012686));
#39321=CARTESIAN_POINT('Ctrl Pts',(0.0546853001230828,0.13225989995725,
-0.11954720910398));
#39322=CARTESIAN_POINT('Ctrl Pts',(-0.080266391393664,0.118492482069505,
-0.112475068195273));
#39323=CARTESIAN_POINT('Ctrl Pts',(-0.143109003210345,-0.00172525958721913,
-0.105402927286567));
#39324=CARTESIAN_POINT('Ctrl Pts',(-0.0773864787151963,-0.120393097438568,
-0.09833078637786));
#39325=CARTESIAN_POINT('Ctrl Pts',(0.0578578832862097,-0.130903100344747,
-0.0912586454691537));
#39326=CARTESIAN_POINT('Ctrl Pts',(0.141124363585093,-0.0238134921719552,
-0.0841865045604471));
#39327=CARTESIAN_POINT('Ctrl Pts',(0.0976086134813589,0.104669637352373,
-0.0771143636517408));
#39328=CARTESIAN_POINT('Ctrl Pts',(-0.0335959010893207,0.139120213170328,
-0.070042222743034));
#39329=CARTESIAN_POINT('Ctrl Pts',(-0.134618961149971,0.0485896016409335,
-0.0629700818343278));
#39330=CARTESIAN_POINT('Ctrl Pts',(-0.114703795973912,-0.0855935473936899,
-0.0558979409256211));
#39331=CARTESIAN_POINT('Ctrl Pts',(0.00825746141212148,-0.142879950729257,
-0.0488258000169147));
#39332=CARTESIAN_POINT('Ctrl Pts',(0.123801572839036,-0.0718105979627093,
-0.0417536591082082));
#39333=CARTESIAN_POINT('Ctrl Pts',(0.128123670011307,0.0637782277226883,
-0.0346815181995017));
#39334=CARTESIAN_POINT('Ctrl Pts',(0.0173471090025586,0.142057483245022,
-0.0276093772907953));
#39335=CARTESIAN_POINT('Ctrl Pts',(-0.109021337153041,0.0927409528906444,
-0.0205372363820887));
#39336=CARTESIAN_POINT('Ctrl Pts',(-0.137433375872942,-0.0399383880652005,
-0.0134650954733823));
#39337=CARTESIAN_POINT('Ctrl Pts',(-0.042407039288203,-0.136648817236048,
-0.00639295456467579));
#39338=CARTESIAN_POINT('Ctrl Pts',(0.0907699169413835,-0.110769430059584,
0.000679186344030648));
#39339=CARTESIAN_POINT('Ctrl Pts',(0.142298180213051,0.0149639330765786,
0.00775132725273722));
#39340=CARTESIAN_POINT('Ctrl Pts',(0.0915728991340969,0.0893085403586358,
0.0124660878585415));
#39341=CARTESIAN_POINT('Ctrl Pts',(0.0560989476895935,0.107773642733835,
0.0148234681614436));
#39342=CARTESIAN_POINT('',(0.067790881553158,-0.100829789141135,0.));
#39343=CARTESIAN_POINT('Ctrl Pts',(0.0679337041871709,-0.100943471330425,
-3.46944695195361E-18));
#39344=CARTESIAN_POINT('Ctrl Pts',(0.0708938339990077,-0.0985098219994332,
-1.14419870693534E-17));
#39345=CARTESIAN_POINT('Ctrl Pts',(0.0737254124732044,-0.095933412712593,
-1.18874367802339E-17));
#39346=CARTESIAN_POINT('Ctrl Pts',(0.0764147067527201,-0.0932157449020129,
-2.08166817117217E-17));
#39347=CARTESIAN_POINT('Ctrl Pts',(0.0810554232312816,-0.0885260663168612,
-3.46280728413895E-17));
#39348=CARTESIAN_POINT('Ctrl Pts',(0.0852732595024775,-0.0834158971715837,
-1.58022670735932E-16));
#39349=CARTESIAN_POINT('Ctrl Pts',(0.0890425996765434,-0.0779563683780291,
-1.92554305833426E-16));
#39350=CARTESIAN_POINT('Ctrl Pts',(0.0911975676765645,-0.0748351033019154,
-2.12296373459876E-16));
#39351=CARTESIAN_POINT('Ctrl Pts',(0.0932003266707534,-0.0716070928834988,
-2.27733886033849E-16));
#39352=CARTESIAN_POINT('Ctrl Pts',(0.095044588107307,-0.0682903407639059,
-2.22044604925031E-16));
#39353=CARTESIAN_POINT('Ctrl Pts',(0.0974021926190729,-0.0640503834527701,
-2.14771734308641E-16));
#39354=CARTESIAN_POINT('Ctrl Pts',(0.0995023637806551,-0.059663325250277,
-3.65192981336413E-17));
#39355=CARTESIAN_POINT('Ctrl Pts',(0.101333546343106,-0.0551577136988226,
-2.42861286636753E-17));
#39356=CARTESIAN_POINT('Ctrl Pts',(0.102909365942388,-0.0512804208853562,
-1.37589051047546E-17));
#39357=CARTESIAN_POINT('Ctrl Pts',(0.10428670233071,-0.0473107226566473,
-9.1622380330981E-17));
#39358=CARTESIAN_POINT('Ctrl Pts',(0.105448892200982,-0.0432949101284721,
-7.97972798949331E-17));
#39359=CARTESIAN_POINT('Ctrl Pts',(0.10781920041327,-0.0351045845560159,
-5.56797639952959E-17));
#39360=CARTESIAN_POINT('Ctrl Pts',(0.109307890077238,-0.0267026497107712,
-1.7069954850417E-18));
#39361=CARTESIAN_POINT('Ctrl Pts',(0.109844464838531,-0.0182481465350914,
3.46944695195361E-18));
#39362=CARTESIAN_POINT('Ctrl Pts',(0.110056959160744,-0.0148999944199391,
5.51942154351163E-18));
#39363=CARTESIAN_POINT('Ctrl Pts',(0.110119567432312,-0.0115436805931865,
-1.07413084515683E-16));
#39364=CARTESIAN_POINT('Ctrl Pts',(0.110025634756424,-0.0081898243220706,
-1.07552855510562E-16));
#39365=CARTESIAN_POINT('Ctrl Pts',(0.109955686614167,-0.0056923332909582,
-1.07656937730521E-16));
#39366=CARTESIAN_POINT('Ctrl Pts',(0.109798760766269,-0.00319835463005472,
-7.98666086115723E-17));
#39367=CARTESIAN_POINT('Ctrl Pts',(0.109553523057914,-0.000720906621662368,
-7.45931094670027E-17));
#39368=CARTESIAN_POINT('Ctrl Pts',(0.10915585786158,0.00329639909887405,
-6.60418671366053E-17));
#39369=CARTESIAN_POINT('Ctrl Pts',(0.108526039512516,0.00727699845794002,
-2.05422639447697E-16));
#39370=CARTESIAN_POINT('Ctrl Pts',(0.107655189039225,0.011202835378149,
-1.795438797636E-16));
#39371=CARTESIAN_POINT('Ctrl Pts',(0.10653757163122,0.0162411098208689,
-1.45609070770046E-16));
#39372=CARTESIAN_POINT('Ctrl Pts',(0.105023066541607,0.0211894402745884,
5.65088878727566E-18));
#39373=CARTESIAN_POINT('Ctrl Pts',(0.103137300132718,0.0260130755751589,
1.73472347597681E-17));
#39374=CARTESIAN_POINT('Ctrl Pts',(0.102077221044583,0.0287246706522717,
2.39223077457933E-17));
#39375=CARTESIAN_POINT('Ctrl Pts',(0.100898998715108,0.0313981896100301,
-1.25490791261462E-16));
#39376=CARTESIAN_POINT('Ctrl Pts',(0.0996086648583684,0.0340221728306018,
-1.14491749414469E-16));
#39377=CARTESIAN_POINT('Ctrl Pts',(0.0960746445368277,0.0412088477957264,
-8.43671136841687E-17));
#39378=CARTESIAN_POINT('Ctrl Pts',(0.0917319904347132,0.0479689262291156,
-1.24597282830284E-17));
#39379=CARTESIAN_POINT('Ctrl Pts',(0.0866841056713385,0.0541743462277911,
3.55618312575245E-17));
#39380=CARTESIAN_POINT('Ctrl Pts',(0.0843006841303288,0.0571043124194059,
5.82358075480046E-17));
#39381=CARTESIAN_POINT('Ctrl Pts',(0.0817595064060622,0.0599101019712312,
-1.67333414005662E-16));
#39382=CARTESIAN_POINT('Ctrl Pts',(0.0790693991906201,0.0625747390717374,
-1.91686944095437E-16));
#39383=CARTESIAN_POINT('Ctrl Pts',(0.0768099707579552,0.0648127750849705,
-2.12141540850814E-16));
#39384=CARTESIAN_POINT('Ctrl Pts',(0.074443867642926,0.066951872301998,
-1.58281656477731E-16));
#39385=CARTESIAN_POINT('Ctrl Pts',(0.0719929118045308,0.0689684036035129,
-1.48318857196017E-16));
#39386=CARTESIAN_POINT('Ctrl Pts',(0.0662253120462789,0.0737137136841467,
-1.24874355329207E-16));
#39387=CARTESIAN_POINT('Ctrl Pts',(0.0599703372361051,0.077803458929088,
-6.83407560972934E-17));
#39388=CARTESIAN_POINT('Ctrl Pts',(0.0533026344467906,0.0811056968029858,
-2.59124319224036E-17));
#39389=CARTESIAN_POINT('Ctrl Pts',(0.0503616242249232,0.0825622577279471,
-7.19802022201604E-18));
#39390=CARTESIAN_POINT('Ctrl Pts',(0.0473401493969273,0.0838649828103428,
-4.46769184301788E-17));
#39391=CARTESIAN_POINT('Ctrl Pts',(0.0442442935173274,0.08499925362115,
-5.11743425413158E-17));
#39392=CARTESIAN_POINT('Ctrl Pts',(-0.121436917850398,-0.000108937277296349,
-0.015489265014994));
#39393=CARTESIAN_POINT('Ctrl Pts',(-0.121530349830317,-0.0115673596937236,
-0.0148145418344567));
#39394=CARTESIAN_POINT('Ctrl Pts',(-0.120038008132328,-0.0230010134756723,
-0.0141398186539195));
#39395=CARTESIAN_POINT('Ctrl Pts',(-0.116860313322169,-0.0339435694343665,
-0.0134650954733823));
#39396=CARTESIAN_POINT('Ctrl Pts',(-0.105757930344696,-0.0721751977888158,
-0.0111077151704802));
#39397=CARTESIAN_POINT('Ctrl Pts',(-0.0740824848164492,-0.104412007512432,
-0.00875033486757794));
#39398=CARTESIAN_POINT('Ctrl Pts',(-0.0360486026807276,-0.116217181178163,
-0.00639295456467575));
#39399=CARTESIAN_POINT('Ctrl Pts',(-0.00166737589937806,-0.126888622803458,
-0.00426196970978384));
#39400=CARTESIAN_POINT('Ctrl Pts',(0.0379096430528989,-0.120864366850511,
-0.00213098485489197));
#39401=CARTESIAN_POINT('Ctrl Pts',(0.0679337041871702,-0.100943471330426,
-5.55111512312578E-17));
#39402=CARTESIAN_POINT('',(0.044346210742013,0.0851009385824475,-0.36));
#39403=CARTESIAN_POINT('Ctrl Pts',(0.0443462107420133,0.0851009385824474,
-0.36));
#39404=CARTESIAN_POINT('Ctrl Pts',(0.0472347321895696,0.084064207117159,
-0.36));
#39405=CARTESIAN_POINT('Ctrl Pts',(0.0500631488172158,0.0828839262856036,
-0.36));
#39406=CARTESIAN_POINT('Ctrl Pts',(0.0528199889486038,0.0815610794408787,
-0.36));
#39407=CARTESIAN_POINT('Ctrl Pts',(0.0566500870458777,0.0797232386733711,
-0.36));
#39408=CARTESIAN_POINT('Ctrl Pts',(0.0603421530117647,0.0776104895128595,
-0.36));
#39409=CARTESIAN_POINT('Ctrl Pts',(0.0638846748154451,0.0752514261108165,
-0.36));
#39410=CARTESIAN_POINT('Ctrl Pts',(0.0667830113424857,0.0733213435293509,
-0.36));
#39411=CARTESIAN_POINT('Ctrl Pts',(0.0695819521300187,0.0712250066688477,
-0.36));
#39412=CARTESIAN_POINT('Ctrl Pts',(0.0722611521682996,0.068988466672373,
-0.36));
#39413=CARTESIAN_POINT('Ctrl Pts',(0.0755956043605516,0.0662049359214967,
-0.36));
#39414=CARTESIAN_POINT('Ctrl Pts',(0.07874992295072,0.0632012229690666,
-0.36));
#39415=CARTESIAN_POINT('Ctrl Pts',(0.0817119391237418,0.0600052355364048,
-0.36));
#39416=CARTESIAN_POINT('Ctrl Pts',(0.0837123729791141,0.0578467863287764,
-0.36));
#39417=CARTESIAN_POINT('Ctrl Pts',(0.0856265812167712,0.0555985564829102,
-0.36));
#39418=CARTESIAN_POINT('Ctrl Pts',(0.0874451964215827,0.0532745140054675,
-0.36));
#39419=CARTESIAN_POINT('Ctrl Pts',(0.0924541421900231,0.0468734882677171,
-0.36));
#39420=CARTESIAN_POINT('Ctrl Pts',(0.0967196599911628,0.0399291210553705,
-0.36));
#39421=CARTESIAN_POINT('Ctrl Pts',(0.100166287100098,0.0326075249336015,
-0.36));
#39422=CARTESIAN_POINT('Ctrl Pts',(0.101810250072491,0.0291152896140918,
-0.36));
#39423=CARTESIAN_POINT('Ctrl Pts',(0.103267542217023,0.0255365320439791,
-0.36));
#39424=CARTESIAN_POINT('Ctrl Pts',(0.1045271934455,0.0218862937333124,-0.36));
#39425=CARTESIAN_POINT('Ctrl Pts',(0.105493737083066,0.0190854274815981,
-0.36));
#39426=CARTESIAN_POINT('Ctrl Pts',(0.106343760940565,0.0162412541306297,
-0.36));
#39427=CARTESIAN_POINT('Ctrl Pts',(0.107068167562164,0.0133774795105766,
-0.36));
#39428=CARTESIAN_POINT('Ctrl Pts',(0.108109295300662,0.00926162095151662,
-0.36));
#39429=CARTESIAN_POINT('Ctrl Pts',(0.108894004138168,0.00509779462631024,
-0.36));
#39430=CARTESIAN_POINT('Ctrl Pts',(0.109410905526584,0.000907155601495218,
-0.36));
#39431=CARTESIAN_POINT('Ctrl Pts',(0.110126047073022,-0.00489066220269337,
-0.36));
#39432=CARTESIAN_POINT('Ctrl Pts',(0.110329285359757,-0.0107397847686723,
-0.36));
#39433=CARTESIAN_POINT('Ctrl Pts',(0.110052890307653,-0.0165912014529204,
-0.36));
#39434=CARTESIAN_POINT('Ctrl Pts',(0.109857463749946,-0.0207284760227993,
-0.36));
#39435=CARTESIAN_POINT('Ctrl Pts',(0.10942034541147,-0.0248732583397424,
-0.36));
#39436=CARTESIAN_POINT('Ctrl Pts',(0.108756338773778,-0.0289741209316136,
-0.36));
#39437=CARTESIAN_POINT('Ctrl Pts',(0.107635003956189,-0.0358994131581975,
-0.36));
#39438=CARTESIAN_POINT('Ctrl Pts',(0.105869233631456,-0.0427137508429052,
-0.36));
#39439=CARTESIAN_POINT('Ctrl Pts',(0.10351308543783,-0.0493365135573982,
-0.36));
#39440=CARTESIAN_POINT('Ctrl Pts',(0.102033997330004,-0.0534939980477481,
-0.36));
#39441=CARTESIAN_POINT('Ctrl Pts',(0.100321758575276,-0.0575761332536055,
-0.36));
#39442=CARTESIAN_POINT('Ctrl Pts',(0.0983851040604554,-0.0615629288935909,
-0.36));
#39443=CARTESIAN_POINT('Ctrl Pts',(0.0970401561620803,-0.0643316377036621,
-0.36));
#39444=CARTESIAN_POINT('Ctrl Pts',(0.095585606598187,-0.0670559753448776,
-0.36));
#39445=CARTESIAN_POINT('Ctrl Pts',(0.0940333458586794,-0.0697137697496087,
-0.36));
#39446=CARTESIAN_POINT('Ctrl Pts',(0.0895102198836054,-0.0774583055756314,
-0.36));
#39447=CARTESIAN_POINT('Ctrl Pts',(0.0841489978738535,-0.0846669728616559,
-0.36));
#39448=CARTESIAN_POINT('Ctrl Pts',(0.0780314158881196,-0.0911818299894396,
-0.36));
#39449=CARTESIAN_POINT('Ctrl Pts',(0.0748243951975507,-0.0945971142722862,
-0.36));
#39450=CARTESIAN_POINT('Ctrl Pts',(0.0714086645011581,-0.0978215835525157,
-0.36));
#39451=CARTESIAN_POINT('Ctrl Pts',(0.0677908815531574,-0.100829789141135,
-0.36));
#39452=CARTESIAN_POINT('Ctrl Pts',(0.044346210742013,0.0851009385824475,
-0.36));
#39453=CARTESIAN_POINT('Ctrl Pts',(0.0190593750035626,0.0980677190231918,
-0.357869015145108));
#39454=CARTESIAN_POINT('Ctrl Pts',(-0.0473907229385778,0.100665673128455,
-0.353380649987314));
#39455=CARTESIAN_POINT('Ctrl Pts',(-0.0930472695895792,0.0423974729753036,
-0.34848489437946));
#39456=CARTESIAN_POINT('Ctrl Pts',(-0.0959255972774781,0.00552313991188578,
-0.345720123626498));
#39457=CARTESIAN_POINT('Ctrl Pts',(-0.0958786240325138,8.20367901696933E-5,
-0.345312733176438));
#39458=CARTESIAN_POINT('Origin',(-1.13809670924099E-17,0.,-0.36));
#39459=CARTESIAN_POINT('',(-0.0659593141366104,0.0695111466142514,-0.36));
#39460=CARTESIAN_POINT('Ctrl Pts',(-0.0374782951795791,-0.115758143579925,
-0.36));
#39461=CARTESIAN_POINT('Ctrl Pts',(-0.0409945590109367,-0.11423469221382,
-0.36));
#39462=CARTESIAN_POINT('Ctrl Pts',(-0.0444266010530333,-0.11253857797051,
-0.36));
#39463=CARTESIAN_POINT('Ctrl Pts',(-0.047760806536058,-0.110667458896572,
-0.36));
#39464=CARTESIAN_POINT('Ctrl Pts',(-0.0535144001878152,-0.107438606061826,
-0.36));
#39465=CARTESIAN_POINT('Ctrl Pts',(-0.058977397035532,-0.103688991136846,
-0.36));
#39466=CARTESIAN_POINT('Ctrl Pts',(-0.0641055674959587,-0.0994799284445121,
-0.36));
#39467=CARTESIAN_POINT('Ctrl Pts',(-0.067037390860062,-0.0970735676502313,
-0.36));
#39468=CARTESIAN_POINT('Ctrl Pts',(-0.0698523243294171,-0.0945226424495796,
-0.36));
#39469=CARTESIAN_POINT('Ctrl Pts',(-0.0725393605821344,-0.0918427255808781,
-0.36));
#39470=CARTESIAN_POINT('Ctrl Pts',(-0.07597432835866,-0.088416858855616,
-0.36));
#39471=CARTESIAN_POINT('Ctrl Pts',(-0.0792023809783025,-0.0847786310744104,
-0.36));
#39472=CARTESIAN_POINT('Ctrl Pts',(-0.0822045421129473,-0.080952298760896,
-0.36));
#39473=CARTESIAN_POINT('Ctrl Pts',(-0.0847880355765678,-0.0776595692642917,
-0.36));
#39474=CARTESIAN_POINT('Ctrl Pts',(-0.0872062056573671,-0.0742233052644298,
-0.36));
#39475=CARTESIAN_POINT('Ctrl Pts',(-0.0894302752531271,-0.0706834112835403,
-0.36));
#39476=CARTESIAN_POINT('Ctrl Pts',(-0.0939663173730785,-0.0634637144592644,
-0.36));
#39477=CARTESIAN_POINT('Ctrl Pts',(-0.0977132205242399,-0.0557975981886947,
-0.36));
#39478=CARTESIAN_POINT('Ctrl Pts',(-0.100559382367918,-0.0478185100843481,
-0.36));
#39479=CARTESIAN_POINT('Ctrl Pts',(-0.101686523476363,-0.0446586201328015,
-0.36));
#39480=CARTESIAN_POINT('Ctrl Pts',(-0.102671833564592,-0.0414495698489802,
-0.36));
#39481=CARTESIAN_POINT('Ctrl Pts',(-0.103505988409046,-0.0381997328206336,
-0.36));
#39482=CARTESIAN_POINT('Ctrl Pts',(-0.104127151899229,-0.0357797023856622,
-0.36));
#39483=CARTESIAN_POINT('Ctrl Pts',(-0.104663738393444,-0.0333390738383591,
-0.36));
#39484=CARTESIAN_POINT('Ctrl Pts',(-0.105110877135444,-0.0308899932766151,
-0.36));
#39485=CARTESIAN_POINT('Ctrl Pts',(-0.105835927921372,-0.0269187252577624,
-0.36));
#39486=CARTESIAN_POINT('Ctrl Pts',(-0.106327704363669,-0.0229187515367,
-0.36));
#39487=CARTESIAN_POINT('Ctrl Pts',(-0.106572694858759,-0.0189049809525404,
-0.36));
#39488=CARTESIAN_POINT('Ctrl Pts',(-0.106887108737049,-0.0137538212086797,
-0.36));
#39489=CARTESIAN_POINT('Ctrl Pts',(-0.106795218220299,-0.00857972307390588,
-0.36));
#39490=CARTESIAN_POINT('Ctrl Pts',(-0.106312078018921,-0.00342315543767976,
-0.36));
#39491=CARTESIAN_POINT('Ctrl Pts',(-0.106040482163523,-0.000524405977197053,
-0.36));
#39492=CARTESIAN_POINT('Ctrl Pts',(-0.105644824844572,0.00237030729199937,
-0.36));
#39493=CARTESIAN_POINT('Ctrl Pts',(-0.105127745376361,0.00524830605462617,
-0.36));
#39494=CARTESIAN_POINT('Ctrl Pts',(-0.103711546170997,0.0131306912802027,
-0.36));
#39495=CARTESIAN_POINT('Ctrl Pts',(-0.101400453867158,0.0208258966356713,
-0.36));
#39496=CARTESIAN_POINT('Ctrl Pts',(-0.0982585663341195,0.0281823183509716,
-0.36));
#39497=CARTESIAN_POINT('Ctrl Pts',(-0.0967750858904105,0.0316557424107343,
-0.36));
#39498=CARTESIAN_POINT('Ctrl Pts',(-0.0951057330825189,0.0350532838824544,
-0.36));
#39499=CARTESIAN_POINT('Ctrl Pts',(-0.0932543133983396,0.0383561915274667,
-0.36));
#39500=CARTESIAN_POINT('Ctrl Pts',(-0.0916992984606194,0.0411303171186509,
-0.36));
#39501=CARTESIAN_POINT('Ctrl Pts',(-0.0900144697478421,0.0438387400352794,
-0.36));
#39502=CARTESIAN_POINT('Ctrl Pts',(-0.0882142913185504,0.0464527333263584,
-0.36));
#39503=CARTESIAN_POINT('Ctrl Pts',(-0.0839781105678046,0.0526039836035903,
-0.36));
#39504=CARTESIAN_POINT('Ctrl Pts',(-0.0790927371523359,0.0582594033379722,
-0.36));
#39505=CARTESIAN_POINT('Ctrl Pts',(-0.0735935572855504,0.0632715851012407,
-0.36));
#39506=CARTESIAN_POINT('Ctrl Pts',(-0.0711679547302304,0.065482380381123,
-0.36));
#39507=CARTESIAN_POINT('Ctrl Pts',(-0.0686226008669145,0.0675674772847997,
-0.36));
#39508=CARTESIAN_POINT('Ctrl Pts',(-0.0659593141366111,0.0695111466142507,
-0.36));
#39509=CARTESIAN_POINT('Origin',(0.,0.,-0.36));
#39510=CARTESIAN_POINT('Origin',(0.,0.,-0.466687266823562));
#39511=CARTESIAN_POINT('Ctrl Pts',(-0.0659593141366105,0.0695111466142513,
-0.36));
#39512=CARTESIAN_POINT('Ctrl Pts',(-0.0847646433244671,0.0516667191265611,
-0.358062422274521));
#39513=CARTESIAN_POINT('Ctrl Pts',(-0.0956440567215446,0.0257261722731044,
-0.356124844549042));
#39514=CARTESIAN_POINT('Ctrl Pts',(-0.095872656538109,-8.6175248921171E-5,
-0.354187266823562));
#39515=CARTESIAN_POINT('Ctrl Pts',(-0.083632211506372,0.0881357089865025,
-0.374823468161444));
#39516=CARTESIAN_POINT('Ctrl Pts',(-0.112642290239959,0.0606079671851011,
-0.372466087858542));
#39517=CARTESIAN_POINT('Ctrl Pts',(-0.14091032653339,-0.0248385438731813,
-0.367751327252738));
#39518=CARTESIAN_POINT('Ctrl Pts',(-0.0567215063177935,-0.131497930301921,
-0.360679186344031));
#39519=CARTESIAN_POINT('Ctrl Pts',(0.0784298127526211,-0.119666359434824,
-0.353607045435325));
#39520=CARTESIAN_POINT('Ctrl Pts',(0.143117945131048,-0.000509442566161793,
-0.346534904526617));
#39521=CARTESIAN_POINT('Ctrl Pts',(0.0792351761535744,0.119198667837268,
-0.339462763617912));
#39522=CARTESIAN_POINT('Ctrl Pts',(-0.0558314673825238,0.131772923774124,
-0.332390622709204));
#39523=CARTESIAN_POINT('Ctrl Pts',(-0.140740043976632,0.025991892761529,
-0.325318481800499));
#39524=CARTESIAN_POINT('Ctrl Pts',(-0.0992120329567224,-0.103153117192596,
-0.318246340891791));
#39525=CARTESIAN_POINT('Ctrl Pts',(0.031445472711221,-0.139621098347674,
-0.311174199983086));
#39526=CARTESIAN_POINT('Ctrl Pts',(0.133853151494439,-0.05066114897936,
-0.304102059074379));
#39527=CARTESIAN_POINT('Ctrl Pts',(0.116010948020474,0.0838133411859342,
-0.297029918165673));
#39528=CARTESIAN_POINT('Ctrl Pts',(-0.00605227524711941,0.142991225558366,
-0.289957777256966));
#39529=CARTESIAN_POINT('Ctrl Pts',(-0.12267829001528,0.0737103367492016,
-0.282885636348259));
#39530=CARTESIAN_POINT('Ctrl Pts',(-0.129093564080224,-0.0617901475075677,
-0.275813495439553));
#39531=CARTESIAN_POINT('Ctrl Pts',(-0.0195347836114904,-0.14177993796111,
-0.268741354530847));
#39532=CARTESIAN_POINT('Ctrl Pts',(0.10757349863316,-0.0943986737283372,
-0.26166921362214));
#39533=CARTESIAN_POINT('Ctrl Pts',(0.138040756604721,0.0377877633064989,
-0.254597072713434));
#39534=CARTESIAN_POINT('Ctrl Pts',(0.0444960554859608,0.136026707539486,
-0.247524931804727));
#39535=CARTESIAN_POINT('Ctrl Pts',(-0.0890226582677377,0.112063070275597,
-0.240452790896021));
#39536=CARTESIAN_POINT('Ctrl Pts',(-0.142565903491056,-0.0125749041412679,
-0.233380649987314));
#39537=CARTESIAN_POINT('Ctrl Pts',(-0.0680319245716216,-0.125915932825319,
-0.226308509078608));
#39538=CARTESIAN_POINT('Ctrl Pts',(0.0676200343668064,-0.126137607550046,
-0.219236368169901));
#39539=CARTESIAN_POINT('Ctrl Pts',(0.142524043916613,-0.0130407793433053,
-0.212164227261195));
#39540=CARTESIAN_POINT('Ctrl Pts',(0.0893884348657091,0.111771520160272,
-0.205092086352488));
#39541=CARTESIAN_POINT('Ctrl Pts',(-0.0440512463399878,0.136171409372038,
-0.198019945443782));
#39542=CARTESIAN_POINT('Ctrl Pts',(-0.137916518725782,0.0382387092123,-0.190947804535075));
#39543=CARTESIAN_POINT('Ctrl Pts',(-0.107881444420903,-0.0940465787220441,
-0.183875663626369));
#39544=CARTESIAN_POINT('Ctrl Pts',(0.0190713051159471,-0.141843048316256,
-0.176803522717662));
#39545=CARTESIAN_POINT('Ctrl Pts',(0.128890926975957,-0.0622116866027405,
-0.169731381808955));
#39546=CARTESIAN_POINT('Ctrl Pts',(0.122918541674049,0.0733089157807597,
-0.162659240900249));
#39547=CARTESIAN_POINT('Ctrl Pts',(0.00651957295741905,0.142970837077603,
-0.155587099991542));
#39548=CARTESIAN_POINT('Ctrl Pts',(-0.115736397526259,0.0841917524929431,
-0.148514959082836));
#39549=CARTESIAN_POINT('Ctrl Pts',(-0.134018023195025,-0.050222848498276,
-0.14144281817413));
#39550=CARTESIAN_POINT('Ctrl Pts',(-0.0319016001457418,-0.139518648620136,
-0.134370677265423));
#39551=CARTESIAN_POINT('Ctrl Pts',(0.0988743262848422,-0.103474787844967,
-0.127298536356717));
#39552=CARTESIAN_POINT('Ctrl Pts',(0.140824326054265,0.0255279206178999,
-0.12022639544801));
#39553=CARTESIAN_POINT('Ctrl Pts',(0.0562616762174438,0.131597078231438,
-0.113154254539304));
#39554=CARTESIAN_POINT('Ctrl Pts',(-0.0788448723527147,0.119443060420805,
-0.106082113630597));
#39555=CARTESIAN_POINT('Ctrl Pts',(-0.143119427000951,-1.51941259976048E-5,
-0.0990099727218907));
#39556=CARTESIAN_POINT('Ctrl Pts',(-0.0788194185783735,-0.119459934035312,
-0.0919378318131843));
#39557=CARTESIAN_POINT('Ctrl Pts',(0.0562896220605368,-0.131584950015693,
-0.0848656909044778));
#39558=CARTESIAN_POINT('Ctrl Pts',(0.140829888105883,-0.0254982124362326,
-0.0777935499957713));
#39559=CARTESIAN_POINT('Ctrl Pts',(0.0988520446283971,0.103496335460187,
-0.0707214090870648));
#39560=CARTESIAN_POINT('Ctrl Pts',(-0.0319308144085461,0.139510902617143,
-0.0636492681783583));
#39561=CARTESIAN_POINT('Ctrl Pts',(-0.134029630703973,0.0501961269752127,
-0.0565771272696519));
#39562=CARTESIAN_POINT('Ctrl Pts',(-0.115716724825556,-0.0842198198972059,
-0.0495049863609454));
#39563=CARTESIAN_POINT('Ctrl Pts',(0.00654668273591539,-0.142962922239377,
-0.0424328454522389));
#39564=CARTESIAN_POINT('Ctrl Pts',(0.122940460166638,-0.0732951485999077,
-0.0353607045435324));
#39565=CARTESIAN_POINT('Ctrl Pts',(0.128865671478577,0.0622627052466987,
-0.028288563634826));
#39566=CARTESIAN_POINT('Ctrl Pts',(0.0190639912086942,0.141802106288977,
-0.0212164227261194));
#39567=CARTESIAN_POINT('Ctrl Pts',(-0.107945428332621,0.0941106766245759,
-0.014144281817413));
#39568=CARTESIAN_POINT('Ctrl Pts',(-0.137820628598294,-0.038446686700647,
-0.00707214090870644));
#39569=CARTESIAN_POINT('Ctrl Pts',(-0.0754254682766369,-0.103308324795554,
-0.00235738030290216));
#39570=CARTESIAN_POINT('Ctrl Pts',(-0.0373723213044952,-0.115609513450726,
0.));
#39571=CARTESIAN_POINT('Ctrl Pts',(-0.0777412457164515,0.0819275215290854,
-0.369882312107629));
#39572=CARTESIAN_POINT('Ctrl Pts',(-0.104707884747748,0.056338805161843,
-0.367524931804727));
#39573=CARTESIAN_POINT('Ctrl Pts',(-0.130984750034776,-0.0230889427375329,
-0.362810171198923));
#39574=CARTESIAN_POINT('Ctrl Pts',(-0.0527261025462999,-0.122235353181203,
-0.355738030290216));
#39575=CARTESIAN_POINT('Ctrl Pts',(0.0729052985072893,-0.111237185831287,
-0.34866588938151));
#39576=CARTESIAN_POINT('Ctrl Pts',(0.133036866279911,-0.000473557962907169,
-0.341593748472803));
#39577=CARTESIAN_POINT('Ctrl Pts',(0.0736539329498896,0.110802437942284,
-0.334521607564097));
#39578=CARTESIAN_POINT('Ctrl Pts',(-0.0518987570257442,0.122490976399911,
-0.32744946665539));
#39579=CARTESIAN_POINT('Ctrl Pts',(-0.130826462003793,0.0241610509325787,
-0.320377325746684));
#39580=CARTESIAN_POINT('Ctrl Pts',(-0.0922236407861768,-0.0958871191571506,
-0.313305184837977));
#39581=CARTESIAN_POINT('Ctrl Pts',(0.0292304863961032,-0.12978633373841,
-0.306233043929271));
#39582=CARTESIAN_POINT('Ctrl Pts',(0.124424675048295,-0.0470926304607176,
-0.299160903020564));
#39583=CARTESIAN_POINT('Ctrl Pts',(0.107839257786109,0.0779096168102174,
-0.292088762111858));
#39584=CARTESIAN_POINT('Ctrl Pts',(-0.00562595928835486,0.13291907270182,
-0.285016621203152));
#39585=CARTESIAN_POINT('Ctrl Pts',(-0.114036959161667,0.0685182574733831,
-0.277944480294445));
#39586=CARTESIAN_POINT('Ctrl Pts',(-0.120000348009553,-0.057437713934847,
-0.270872339385738));
#39587=CARTESIAN_POINT('Ctrl Pts',(-0.0181587738193776,-0.131793106940118,
-0.263800198477032));
#39588=CARTESIAN_POINT('Ctrl Pts',(0.0999961335373955,-0.0877493295637964,
-0.256728057568325));
#39589=CARTESIAN_POINT('Ctrl Pts',(0.128317309620287,0.0351260326538398,
-0.249655916659619));
#39590=CARTESIAN_POINT('Ctrl Pts',(0.0413617997257353,0.126445128071512,
-0.242583775750912));
#39591=CARTESIAN_POINT('Ctrl Pts',(-0.0827519950276166,0.104169464433825,
-0.235511634842206));
#39592=CARTESIAN_POINT('Ctrl Pts',(-0.132523709877523,-0.0116891410031967,
-0.228439493933499));
#39593=CARTESIAN_POINT('Ctrl Pts',(-0.0632398267297108,-0.117046545787487,
-0.221367353024793));
#39594=CARTESIAN_POINT('Ctrl Pts',(0.0628569496415179,-0.117252605975705,
-0.214295212116086));
#39595=CARTESIAN_POINT('Ctrl Pts',(0.132484798847864,-0.0121222004416881,
-0.20722307120738));
#39596=CARTESIAN_POINT('Ctrl Pts',(0.0830920067033574,0.103898450804675,
-0.200150930298674));
#39597=CARTESIAN_POINT('Ctrl Pts',(-0.0409483224722811,0.126579637257834,
-0.193078789389967));
#39598=CARTESIAN_POINT('Ctrl Pts',(-0.12820182292802,0.0355452144001576,
-0.186006648481261));
#39599=CARTESIAN_POINT('Ctrl Pts',(-0.100282387944889,-0.0874220357626795,
-0.178934507572554));
#39600=CARTESIAN_POINT('Ctrl Pts',(0.0177279422658734,-0.131851771867642,
-0.171862366663848));
#39601=CARTESIAN_POINT('Ctrl Pts',(0.119811984451657,-0.05782956025562,
-0.164790225755141));
#39602=CARTESIAN_POINT('Ctrl Pts',(0.11426028774406,0.0681451121794678,
-0.157718084846435));
#39603=CARTESIAN_POINT('Ctrl Pts',(0.0060603410351095,0.132900120364386,
-0.150645943937728));
#39604=CARTESIAN_POINT('Ctrl Pts',(-0.107584046342482,0.078261373219263,
-0.143573803029022));
#39605=CARTESIAN_POINT('Ctrl Pts',(-0.124577933358174,-0.046685203408583,
-0.136501662120315));
#39606=CARTESIAN_POINT('Ctrl Pts',(-0.0296544846896594,-0.129691100462874,
-0.129429521211609));
#39607=CARTESIAN_POINT('Ctrl Pts',(0.0919097218201968,-0.0961861316641179,
-0.122357380302902));
#39608=CARTESIAN_POINT('Ctrl Pts',(0.130904807339743,0.0237297605030454,
-0.115285239394196));
#39609=CARTESIAN_POINT('Ctrl Pts',(0.0522986623988346,0.122327517233929,
-0.108213098485489));
#39610=CARTESIAN_POINT('Ctrl Pts',(-0.0732911217418617,0.111029615767021,
-0.101140957576783));
#39611=CARTESIAN_POINT('Ctrl Pts',(-0.133038243768442,-1.41238676029155E-5,
-0.0940688166680761));
#39612=CARTESIAN_POINT('Ctrl Pts',(-0.0732674609048485,-0.111045300821714,
-0.0869966757593698));
#39613=CARTESIAN_POINT('Ctrl Pts',(0.0523246397658751,-0.122316243317057,
-0.0799245348506631));
#39614=CARTESIAN_POINT('Ctrl Pts',(0.130909977606244,-0.0237021449347227,
-0.0728523939419569));
#39615=CARTESIAN_POINT('Ctrl Pts',(0.0918890096604021,0.0962061614877861,
-0.0657802530332501));
#39616=CARTESIAN_POINT('Ctrl Pts',(-0.0296816411302489,0.129683900080257,
-0.058708112124544));
#39617=CARTESIAN_POINT('Ctrl Pts',(-0.124588723246293,0.0466603641217457,
-0.0516359712158372));
#39618=CARTESIAN_POINT('Ctrl Pts',(-0.107565759366307,-0.0782874635848309,
-0.0445638303071309));
#39619=CARTESIAN_POINT('Ctrl Pts',(0.0060855412290717,-0.132892763039114,
-0.0374916893984244));
#39620=CARTESIAN_POINT('Ctrl Pts',(0.114280662320881,-0.0681323147444817,
-0.0304195484897179));
#39621=CARTESIAN_POINT('Ctrl Pts',(0.119788507925182,0.0578769851994863,
-0.0233474075810114));
#39622=CARTESIAN_POINT('Ctrl Pts',(0.017721143542622,0.131813713754082,
-0.0162752666723049));
#39623=CARTESIAN_POINT('Ctrl Pts',(-0.100341864896571,0.0874816186757801,
-0.00920312576359841));
#39624=CARTESIAN_POINT('Ctrl Pts',(-0.128112687201144,-0.0357385421710475,
-0.0021309848548919));
#39625=CARTESIAN_POINT('Ctrl Pts',(-0.0701125769240916,-0.0960313940983636,
0.00258377575091239));
#39626=CARTESIAN_POINT('Ctrl Pts',(-0.0347398539533484,-0.10746609984895,
0.00494115605381455));
#39627=CARTESIAN_POINT('Ctrl Pts',(-0.071850279926531,0.0757193340716684,
-0.364941156053815));
#39628=CARTESIAN_POINT('Ctrl Pts',(-0.0967734792555375,0.0520696431385851,
-0.362583775750912));
#39629=CARTESIAN_POINT('Ctrl Pts',(-0.121059173536162,-0.0213393416018847,
-0.357869015145108));
#39630=CARTESIAN_POINT('Ctrl Pts',(-0.0487306987748063,-0.112972776060485,
-0.350796874236402));
#39631=CARTESIAN_POINT('Ctrl Pts',(0.0673807842619576,-0.10280801222775,
-0.343724733327695));
#39632=CARTESIAN_POINT('Ctrl Pts',(0.122955787428773,-0.00043767335965257,
-0.336652592418989));
#39633=CARTESIAN_POINT('Ctrl Pts',(0.0680726897462049,0.102406208047299,
-0.329580451510282));
#39634=CARTESIAN_POINT('Ctrl Pts',(-0.0479660466689646,0.113209029025698,
-0.322508310601576));
#39635=CARTESIAN_POINT('Ctrl Pts',(-0.120912880030953,0.0223302091036286,
-0.315436169692869));
#39636=CARTESIAN_POINT('Ctrl Pts',(-0.085235248615631,-0.0886211211217054,
-0.308364028784163));
#39637=CARTESIAN_POINT('Ctrl Pts',(0.0270155000809852,-0.119951569129147,
-0.301291887875456));
#39638=CARTESIAN_POINT('Ctrl Pts',(0.11499619860215,-0.0435241119420751,
-0.29421974696675));
#39639=CARTESIAN_POINT('Ctrl Pts',(0.0996675675517452,0.0720058924345007,
-0.287147606058044));
#39640=CARTESIAN_POINT('Ctrl Pts',(-0.00519964332959026,0.122846919845274,
-0.280075465149336));
#39641=CARTESIAN_POINT('Ctrl Pts',(-0.105395628308053,0.0633261781975646,
-0.273003324240631));
#39642=CARTESIAN_POINT('Ctrl Pts',(-0.110907131938881,-0.0530852803621263,
-0.265931183331924));
#39643=CARTESIAN_POINT('Ctrl Pts',(-0.0167827640272648,-0.121806275919127,
-0.258859042423217));
#39644=CARTESIAN_POINT('Ctrl Pts',(0.0924187684416306,-0.0810999853992555,
-0.251786901514511));
#39645=CARTESIAN_POINT('Ctrl Pts',(0.118593862635852,0.0324643020011807,
-0.244714760605804));
#39646=CARTESIAN_POINT('Ctrl Pts',(0.03822754396551,0.116863548603539,-0.237642619697098));
#39647=CARTESIAN_POINT('Ctrl Pts',(-0.0764813317874957,0.0962758585920524,
-0.230570478788392));
#39648=CARTESIAN_POINT('Ctrl Pts',(-0.122481516263989,-0.0108033778651255,
-0.223498337879685));
#39649=CARTESIAN_POINT('Ctrl Pts',(-0.0584477288878,-0.108177158749654,
-0.216426196970979));
#39650=CARTESIAN_POINT('Ctrl Pts',(0.0580938649162294,-0.108367604401363,
-0.209354056062272));
#39651=CARTESIAN_POINT('Ctrl Pts',(0.122445553779115,-0.0112036215400709,
-0.202281915153565));
#39652=CARTESIAN_POINT('Ctrl Pts',(0.0767955785410057,0.0960253814490789,
-0.195209774244859));
#39653=CARTESIAN_POINT('Ctrl Pts',(-0.0378453986045744,0.116987865143631,
-0.188137633336152));
#39654=CARTESIAN_POINT('Ctrl Pts',(-0.118487127130257,0.0328517195880153,
-0.181065492427446));
#39655=CARTESIAN_POINT('Ctrl Pts',(-0.0926833314688766,-0.080797492803315,
-0.173993351518739));
#39656=CARTESIAN_POINT('Ctrl Pts',(0.0163845794157999,-0.121860495419028,
-0.166921210610033));
#39657=CARTESIAN_POINT('Ctrl Pts',(0.110733041927356,-0.0534474339084993,
-0.159849069701326));
#39658=CARTESIAN_POINT('Ctrl Pts',(0.10560203381407,0.0629813085781758,
-0.15277692879262));
#39659=CARTESIAN_POINT('Ctrl Pts',(0.00560110911279988,0.12282940365117,
-0.145704787883913));
#39660=CARTESIAN_POINT('Ctrl Pts',(-0.0994316951587051,0.0723309939455828,
-0.138632646975207));
#39661=CARTESIAN_POINT('Ctrl Pts',(-0.115137843521322,-0.0431475583188898,
-0.1315605060665));
#39662=CARTESIAN_POINT('Ctrl Pts',(-0.027407369233577,-0.119863552305612,
-0.124488365157794));
#39663=CARTESIAN_POINT('Ctrl Pts',(0.0849451173555514,-0.0888974754832685,
-0.117416224249088));
#39664=CARTESIAN_POINT('Ctrl Pts',(0.120985288625221,0.021931600388191,
-0.110344083340381));
#39665=CARTESIAN_POINT('Ctrl Pts',(0.0483356485802257,0.113057956236419,
-0.103271942431675));
#39666=CARTESIAN_POINT('Ctrl Pts',(-0.0677373711310089,0.102616171113238,
-0.0961998015229683));
#39667=CARTESIAN_POINT('Ctrl Pts',(-0.122957060535933,-1.30536092081419E-5,
-0.0891276606142616));
#39668=CARTESIAN_POINT('Ctrl Pts',(-0.0677155032313236,-0.102630667608116,
-0.0820555197055553));
#39669=CARTESIAN_POINT('Ctrl Pts',(0.0483596574712134,-0.11304753661842,
-0.0749833787968486));
#39670=CARTESIAN_POINT('Ctrl Pts',(0.120990067106604,-0.0219060774332128,
-0.0679112378881423));
#39671=CARTESIAN_POINT('Ctrl Pts',(0.0849259746924071,0.088915987515385,
-0.0608390969794358));
#39672=CARTESIAN_POINT('Ctrl Pts',(-0.0274324678519518,0.11985689754337,
-0.0537669560707292));
#39673=CARTESIAN_POINT('Ctrl Pts',(-0.115147815788613,0.043124601268279,
-0.0466948151620228));
#39674=CARTESIAN_POINT('Ctrl Pts',(-0.0994147939070581,-0.0723551072724562,
-0.0396226742533162));
#39675=CARTESIAN_POINT('Ctrl Pts',(0.00562439972222807,-0.122822603838851,
-0.0325505333446099));
#39676=CARTESIAN_POINT('Ctrl Pts',(0.105620864475125,-0.0629694808890559,
-0.0254783924359033));
#39677=CARTESIAN_POINT('Ctrl Pts',(0.110711344371787,0.0534912651522741,
-0.0184062515271969));
#39678=CARTESIAN_POINT('Ctrl Pts',(0.0163782958765497,0.121825321219186,
-0.0113341106184903));
#39679=CARTESIAN_POINT('Ctrl Pts',(-0.092738301460522,0.0808525607269844,
-0.00426196970978388));
#39680=CARTESIAN_POINT('Ctrl Pts',(-0.118404745803993,-0.0330303976414481,
0.00281017119892266));
#39681=CARTESIAN_POINT('Ctrl Pts',(-0.0647996855715466,-0.0887544634011735,
0.00752493180472693));
#39682=CARTESIAN_POINT('Ctrl Pts',(-0.0321073866022016,-0.0993226862471739,
0.00988231210762909));
#39683=CARTESIAN_POINT('Ctrl Pts',(-0.0659593141366105,0.0695111466142513,
-0.36));
#39684=CARTESIAN_POINT('Ctrl Pts',(-0.0888390737633265,0.047800481115327,
-0.357642619697098));
#39685=CARTESIAN_POINT('Ctrl Pts',(-0.111133597037548,-0.0195897404662363,
-0.352927859091294));
#39686=CARTESIAN_POINT('Ctrl Pts',(-0.0447352950033125,-0.103710198939767,
-0.345855718182587));
#39687=CARTESIAN_POINT('Ctrl Pts',(0.0618562700166257,-0.0943788386242131,
-0.338783577273881));
#39688=CARTESIAN_POINT('Ctrl Pts',(0.112874708577635,-0.000401788756397879,
-0.331711436365174));
#39689=CARTESIAN_POINT('Ctrl Pts',(0.06249144654252,0.0940099781523149,
-0.324639295456468));
#39690=CARTESIAN_POINT('Ctrl Pts',(-0.0440333363121848,0.103927081651485,
-0.317567154547761));
#39691=CARTESIAN_POINT('Ctrl Pts',(-0.110999298058114,0.0204993672746782,
-0.310495013639055));
#39692=CARTESIAN_POINT('Ctrl Pts',(-0.0782468564450852,-0.0813551230862599,
-0.303422872730348));
#39693=CARTESIAN_POINT('Ctrl Pts',(0.0248005137658673,-0.110116804519884,
-0.296350731821642));
#39694=CARTESIAN_POINT('Ctrl Pts',(0.105567722156006,-0.0399555934234326,
-0.289278590912935));
#39695=CARTESIAN_POINT('Ctrl Pts',(0.0914958773173812,0.0661021680587838,
-0.282206450004229));
#39696=CARTESIAN_POINT('Ctrl Pts',(-0.00477332737082577,0.112774766988728,
-0.275134309095522));
#39697=CARTESIAN_POINT('Ctrl Pts',(-0.0967542974544388,0.058134098921746,
-0.268062168186816));
#39698=CARTESIAN_POINT('Ctrl Pts',(-0.101813915868209,-0.0487328467894054,
-0.260990027278109));
#39699=CARTESIAN_POINT('Ctrl Pts',(-0.0154067542351519,-0.111819444898135,
-0.253917886369403));
#39700=CARTESIAN_POINT('Ctrl Pts',(0.0848414033458655,-0.0744506412347145,
-0.246845745460696));
#39701=CARTESIAN_POINT('Ctrl Pts',(0.108870415651418,0.0298025713485215,
-0.23977360455199));
#39702=CARTESIAN_POINT('Ctrl Pts',(0.0350932882052845,0.107281969135566,
-0.232701463643283));
#39703=CARTESIAN_POINT('Ctrl Pts',(-0.0702106685473747,0.08838225275028,
-0.225629322734577));
#39704=CARTESIAN_POINT('Ctrl Pts',(-0.112439322650456,-0.0099176147270544,
-0.21855718182587));
#39705=CARTESIAN_POINT('Ctrl Pts',(-0.0536556310458891,-0.0993077717118213,
-0.211485040917164));
#39706=CARTESIAN_POINT('Ctrl Pts',(0.0533307801909408,-0.0994826028270216,
-0.204412900008458));
#39707=CARTESIAN_POINT('Ctrl Pts',(0.112406308710366,-0.0102850426384537,
-0.197340759099751));
#39708=CARTESIAN_POINT('Ctrl Pts',(0.0704991503786541,0.0881523120934825,
-0.190268618191045));
#39709=CARTESIAN_POINT('Ctrl Pts',(-0.0347424747368677,0.107396093029428,
-0.183196477282338));
#39710=CARTESIAN_POINT('Ctrl Pts',(-0.108772431332495,0.0301582247758729,
-0.176124336373632));
#39711=CARTESIAN_POINT('Ctrl Pts',(-0.0850842749928634,-0.0741729498439504,
-0.169052195464925));
#39712=CARTESIAN_POINT('Ctrl Pts',(0.0150412165657262,-0.111869218970413,
-0.161980054556218));
#39713=CARTESIAN_POINT('Ctrl Pts',(0.101654099403055,-0.0490653075613788,
-0.154907913647512));
#39714=CARTESIAN_POINT('Ctrl Pts',(0.09694377988408,0.0578175049768839,
-0.147835772738805));
#39715=CARTESIAN_POINT('Ctrl Pts',(0.00514187719049035,0.112758686937953,
-0.140763631830099));
#39716=CARTESIAN_POINT('Ctrl Pts',(-0.0912793439749284,0.0664006146719027,
-0.133691490921393));
#39717=CARTESIAN_POINT('Ctrl Pts',(-0.105697753684471,-0.0396099132291967,
-0.126619350012686));
#39718=CARTESIAN_POINT('Ctrl Pts',(-0.0251602537774947,-0.11003600414835,
-0.11954720910398));
#39719=CARTESIAN_POINT('Ctrl Pts',(0.0779805128909062,-0.081608819302419,
-0.112475068195273));
#39720=CARTESIAN_POINT('Ctrl Pts',(0.111065769910699,0.0201334402733364,
-0.105402927286567));
#39721=CARTESIAN_POINT('Ctrl Pts',(0.0443726347616168,0.10378839523891,
-0.0983307863778601));
#39722=CARTESIAN_POINT('Ctrl Pts',(-0.0621836205201562,0.0942027264594536,
-0.0912586454691536));
#39723=CARTESIAN_POINT('Ctrl Pts',(-0.112875877303425,-1.19833508133767E-5,
-0.0841865045604471));
#39724=CARTESIAN_POINT('Ctrl Pts',(-0.0621635455577987,-0.0942160343945172,
-0.0771143636517407));
#39725=CARTESIAN_POINT('Ctrl Pts',(0.0443946751765518,-0.103778829919784,
-0.0700422227430341));
#39726=CARTESIAN_POINT('Ctrl Pts',(0.111070156606965,-0.0201100099317029,
-0.0629700818343277));
#39727=CARTESIAN_POINT('Ctrl Pts',(0.077962939724412,0.0816258135429839,
-0.0558979409256211));
#39728=CARTESIAN_POINT('Ctrl Pts',(-0.0251832945736545,0.110029895006483,
-0.0488258000169148));
#39729=CARTESIAN_POINT('Ctrl Pts',(-0.105706908330933,0.0395888384148121,
-0.0417536591082082));
#39730=CARTESIAN_POINT('Ctrl Pts',(-0.0912638284478091,-0.0664227509600812,
-0.0346815181995017));
#39731=CARTESIAN_POINT('Ctrl Pts',(0.00516325821538433,-0.112752444638587,
-0.0276093772907953));
#39732=CARTESIAN_POINT('Ctrl Pts',(0.0969610666293677,-0.0578066470336301,
-0.0205372363820888));
#39733=CARTESIAN_POINT('Ctrl Pts',(0.101634180818392,0.0491055451050618,
-0.0134650954733823));
#39734=CARTESIAN_POINT('Ctrl Pts',(0.0150354482104775,0.11183692868429,
-0.00639295456467577));
#39735=CARTESIAN_POINT('Ctrl Pts',(-0.0851347380244728,0.0742235027781887,
0.000679186344030675));
#39736=CARTESIAN_POINT('Ctrl Pts',(-0.108696804406843,-0.0303222531118487,
0.0077513272527372));
#39737=CARTESIAN_POINT('Ctrl Pts',(-0.0594867942190013,-0.0814775327039834,
0.0124660878585415));
#39738=CARTESIAN_POINT('Ctrl Pts',(-0.0294749192510548,-0.0911792726453979,
0.0148234681614436));
#39739=CARTESIAN_POINT('',(-0.0373723213044952,-0.115609513450726,0.));
#39740=CARTESIAN_POINT('Ctrl Pts',(-0.0660853196898438,0.0695807828091147,
-3.64291929955129E-17));
#39741=CARTESIAN_POINT('Ctrl Pts',(-0.0685761827410638,0.0677880282189264,
-4.43191730826681E-17));
#39742=CARTESIAN_POINT('Ctrl Pts',(-0.0709697016741088,0.0658738526129303,
-1.8031305068503E-16));
#39743=CARTESIAN_POINT('Ctrl Pts',(-0.0732551202417263,0.0638423633381038,
-1.14491749414469E-16));
#39744=CARTESIAN_POINT('Ctrl Pts',(-0.0764302659566424,0.0610200031117285,
-2.31649688122036E-17));
#39745=CARTESIAN_POINT('Ctrl Pts',(-0.0793969518401287,0.0579714320251634,
1.14889233545085E-16));
#39746=CARTESIAN_POINT('Ctrl Pts',(-0.0821519934974501,0.0547273093807734,
6.59194920871187E-17));
#39747=CARTESIAN_POINT('Ctrl Pts',(-0.0844060535136914,0.0520731037279949,
2.58544949090369E-17));
#39748=CARTESIAN_POINT('Ctrl Pts',(-0.0865187418317461,0.0492864813759394,
-3.25476132089893E-17));
#39749=CARTESIAN_POINT('Ctrl Pts',(-0.0884776822274611,0.0463980921212896,
-4.33680868994202E-17));
#39750=CARTESIAN_POINT('Ctrl Pts',(-0.0909157026986048,0.0428033160133124,
-5.68348245410797E-17));
#39751=CARTESIAN_POINT('Ctrl Pts',(-0.093119879899582,0.0390465411034455,
1.20977856733227E-17));
#39752=CARTESIAN_POINT('Ctrl Pts',(-0.0950862089588394,0.0351579474418293,
-1.90819582357449E-17));
#39753=CARTESIAN_POINT('Ctrl Pts',(-0.0964142002011996,0.0325317245808024,
-4.01396884540584E-17));
#39754=CARTESIAN_POINT('Ctrl Pts',(-0.0976345593006655,0.0298429662492554,
1.52954116439559E-16));
#39755=CARTESIAN_POINT('Ctrl Pts',(-0.0987421319932224,0.0271076808973025,
1.43982048506075E-16));
#39756=CARTESIAN_POINT('Ctrl Pts',(-0.101792681749017,0.0195739775850942,
1.1927058728336E-16));
#39757=CARTESIAN_POINT('Ctrl Pts',(-0.103978837473498,0.0117228968643841,
-3.41615823321009E-18));
#39758=CARTESIAN_POINT('Ctrl Pts',(-0.105273847015717,0.00373491552187747,
3.12250225675825E-17));
#39759=CARTESIAN_POINT('Ctrl Pts',(-0.105891535872104,-7.51622415972098E-5,
4.77480447192829E-17));
#39760=CARTESIAN_POINT('Ctrl Pts',(-0.106305937424425,-0.00391695734714767,
-5.36856847393132E-17));
#39761=CARTESIAN_POINT('Ctrl Pts',(-0.106510652645819,-0.00777298745154552,
-7.11236625150491E-17));
#39762=CARTESIAN_POINT('Ctrl Pts',(-0.106667735066978,-0.010731802828013,
-8.45042003688641E-17));
#39763=CARTESIAN_POINT('Ctrl Pts',(-0.106700871473537,-0.0137001311918125,
-5.41871049115136E-17));
#39764=CARTESIAN_POINT('Ctrl Pts',(-0.106607850951963,-0.0166526766578767,
-3.46944695195361E-17));
#39765=CARTESIAN_POINT('Ctrl Pts',(-0.106474162175508,-0.0208960649351067,
-6.67972039362386E-18));
#39766=CARTESIAN_POINT('Ctrl Pts',(-0.106080766254757,-0.0251148848213788,
1.19106406122488E-16));
#39767=CARTESIAN_POINT('Ctrl Pts',(-0.105422546985642,-0.0292856618406229,
1.24032728532342E-16));
#39768=CARTESIAN_POINT('Ctrl Pts',(-0.104511890193629,-0.0350559979562071,
1.30930489878205E-16));
#39769=CARTESIAN_POINT('Ctrl Pts',(-0.103095019822919,-0.0407345534069762,
6.21935622857477E-17));
#39770=CARTESIAN_POINT('Ctrl Pts',(-0.101216464695186,-0.0462831105067708,
7.45931094670027E-17));
#39771=CARTESIAN_POINT('Ctrl Pts',(-0.0998882206379262,-0.0502062522263654,
8.33602862259234E-17));
#39772=CARTESIAN_POINT('Ctrl Pts',(-0.0983255778215935,-0.0540699920418813,
1.71835757213981E-16));
#39773=CARTESIAN_POINT('Ctrl Pts',(-0.0965569416166795,-0.057828974809559,
1.33573707650214E-16));
#39774=CARTESIAN_POINT('Ctrl Pts',(-0.0935701769319145,-0.0641769150755935,
6.89590977681626E-17));
#39775=CARTESIAN_POINT('Ctrl Pts',(-0.0899945245784868,-0.0702405695530934,
5.19776018937355E-17));
#39776=CARTESIAN_POINT('Ctrl Pts',(-0.085904169907901,-0.0759573404259926,
5.85469173142172E-17));
#39777=CARTESIAN_POINT('Ctrl Pts',(-0.0833364217251236,-0.0795460825284323,
6.2670850100373E-17));
#39778=CARTESIAN_POINT('Ctrl Pts',(-0.080565323852325,-0.08299812931733,
-1.25005049996683E-16));
#39779=CARTESIAN_POINT('Ctrl Pts',(-0.0776047828277375,-0.0862966723715114,
-1.50487261540988E-16));
#39780=CARTESIAN_POINT('Ctrl Pts',(-0.0755487774768718,-0.0885874098121124,
-1.68183879440172E-16));
#39781=CARTESIAN_POINT('Ctrl Pts',(-0.0733996466487082,-0.0908052846402178,
-4.16397669135319E-17));
#39782=CARTESIAN_POINT('Ctrl Pts',(-0.0711749316358312,-0.0929322610972621,
-3.16587034365767E-17));
#39783=CARTESIAN_POINT('Ctrl Pts',(-0.0646923432322698,-0.0991300495039903,
-2.57492147960364E-18));
#39784=CARTESIAN_POINT('Ctrl Pts',(-0.0575518306578732,-0.104581716780799,
1.24711580510287E-17));
#39785=CARTESIAN_POINT('Ctrl Pts',(-0.0498754978577729,-0.109157967797725,
1.78893358460108E-17));
#39786=CARTESIAN_POINT('Ctrl Pts',(-0.0458513303512718,-0.111556977992237,
2.07297097061342E-17));
#39787=CARTESIAN_POINT('Ctrl Pts',(-0.0416791333594398,-0.113715035869443,
-1.34694802438231E-17));
#39788=CARTESIAN_POINT('Ctrl Pts',(-0.0373723213044952,-0.115609513450726,
-8.67361737988404E-19));
#39789=CARTESIAN_POINT('Ctrl Pts',(-0.0373723213044952,-0.115609513450726,
-8.67361737988404E-19));
#39790=CARTESIAN_POINT('Ctrl Pts',(-0.0754254682766369,-0.103308324795554,
-0.00235738030290216));
#39791=CARTESIAN_POINT('Ctrl Pts',(-0.106623048437465,-0.0708775057481003,
-0.00471476060580431));
#39792=CARTESIAN_POINT('Ctrl Pts',(-0.117242638473601,-0.0325692023368365,
-0.00707214090870647));
#39793=CARTESIAN_POINT('Ctrl Pts',(-0.120153648675821,-0.0220682449853316,
-0.00771833893413964));
#39794=CARTESIAN_POINT('Ctrl Pts',(-0.121518425988536,-0.0111256526842618,
-0.0083645369595728));
#39795=CARTESIAN_POINT('Ctrl Pts',(-0.12142737051279,-0.000153818344799855,
-0.00901073498500596));
#39796=CARTESIAN_POINT('Origin',(0.,0.,-0.19));
#39797=CARTESIAN_POINT('Origin',(0.,0.,0.));
#39798=CARTESIAN_POINT('Origin',(0.,0.,0.360944059763209));
#39799=CARTESIAN_POINT('',(0.,0.,0.321888119526417));
#39800=CARTESIAN_POINT('',(-0.13,-1.59204083889156E-17,0.4));
#39801=CARTESIAN_POINT('',(-0.065,-7.9602041944578E-18,0.360944059763209));
#39802=CARTESIAN_POINT('Origin',(0.,0.,0.4));
#39803=CARTESIAN_POINT('Origin',(0.,0.,0.675));
#39804=CARTESIAN_POINT('',(-0.13,-1.59204083889156E-17,0.95));
#39805=CARTESIAN_POINT('',(-0.13,-1.59204083889156E-17,0.675));
#39806=CARTESIAN_POINT('Origin',(0.,0.,0.95));
#39807=CARTESIAN_POINT('Origin',(0.,0.,1.));
#39808=CARTESIAN_POINT('',(-0.18,2.20436423846524E-17,1.));
#39809=CARTESIAN_POINT('',(-0.18,-2.20436423846524E-17,1.));
#39810=CARTESIAN_POINT('Origin',(0.,0.,1.));
#39811=CARTESIAN_POINT('Origin',(0.,0.,0.0275));
#39812=CARTESIAN_POINT('',(0.144337567297406,0.25,0.0336751345948129));
#39813=CARTESIAN_POINT('',(0.0502493781056046,0.25,0.));
#39814=CARTESIAN_POINT('Ctrl Pts',(0.144337567297406,0.25,0.0336751345948129));
#39815=CARTESIAN_POINT('Ctrl Pts',(0.094379570415743,0.25,0.00869613615398113));
#39816=CARTESIAN_POINT('Ctrl Pts',(0.0502493781056046,0.25,-6.93889390390723E-18));
#39817=CARTESIAN_POINT('',(0.191381661893307,0.168517237963823,0.));
#39818=CARTESIAN_POINT('Ctrl Pts',(0.191381661893307,0.168517237963823,
1.73472347597681E-17));
#39819=CARTESIAN_POINT('Ctrl Pts',(0.169316565738238,0.206735105578296,
0.00869613615398118));
#39820=CARTESIAN_POINT('Ctrl Pts',(0.144337567297406,0.25,0.0336751345948129));
#39821=CARTESIAN_POINT('Origin',(0.,0.,0.));
#39822=CARTESIAN_POINT('Origin',(0.,0.,0.0275));
#39823=CARTESIAN_POINT('',(-0.144337567297406,0.25,0.0336751345948129));
#39824=CARTESIAN_POINT('',(-0.191381661893307,0.168517237963823,1.73472347597681E-17));
#39825=CARTESIAN_POINT('Ctrl Pts',(-0.144337567297406,0.25,0.0336751345948129));
#39826=CARTESIAN_POINT('Ctrl Pts',(-0.169316565738238,0.206735105578296,
0.00869613615398114));
#39827=CARTESIAN_POINT('Ctrl Pts',(-0.191381661893307,0.168517237963823,
1.73472347597681E-17));
#39828=CARTESIAN_POINT('',(-0.0502493781056045,0.25,1.04083408558608E-17));
#39829=CARTESIAN_POINT('Ctrl Pts',(-0.0502493781056045,0.25,3.46944695195361E-18));
#39830=CARTESIAN_POINT('Ctrl Pts',(-0.094379570415743,0.25,0.00869613615398118));
#39831=CARTESIAN_POINT('Ctrl Pts',(-0.144337567297406,0.25,0.0336751345948129));
#39832=CARTESIAN_POINT('Origin',(0.,0.,0.));
#39833=CARTESIAN_POINT('Origin',(0.,0.,0.0275));
#39834=CARTESIAN_POINT('',(-0.288675134594813,3.53525079574969E-17,0.0336751345948129));
#39835=CARTESIAN_POINT('',(-0.241631039998912,-0.081482762036177,-1.73472347597681E-17));
#39836=CARTESIAN_POINT('Ctrl Pts',(-0.288675134594813,3.53525079574969E-17,
0.0336751345948129));
#39837=CARTESIAN_POINT('Ctrl Pts',(-0.263696136153981,-0.0432648944217043,
0.00869613615398115));
#39838=CARTESIAN_POINT('Ctrl Pts',(-0.241631039998912,-0.081482762036177,
1.04083408558608E-17));
#39839=CARTESIAN_POINT('',(-0.241631039998912,0.081482762036177,1.73472347597681E-17));
#39840=CARTESIAN_POINT('Ctrl Pts',(-0.241631039998912,0.081482762036177,
1.73472347597681E-17));
#39841=CARTESIAN_POINT('Ctrl Pts',(-0.263696136153981,0.0432648944217042,
0.00869613615398121));
#39842=CARTESIAN_POINT('Ctrl Pts',(-0.288675134594813,3.53525079574969E-17,
0.0336751345948129));
#39843=CARTESIAN_POINT('Origin',(0.,0.,0.));
#39844=CARTESIAN_POINT('Origin',(0.,0.,0.0275));
#39845=CARTESIAN_POINT('',(-0.144337567297407,-0.25,0.0336751345948129));
#39846=CARTESIAN_POINT('',(-0.0502493781056046,-0.25,-2.42861286636753E-17));
#39847=CARTESIAN_POINT('Ctrl Pts',(-0.144337567297407,-0.25,0.0336751345948129));
#39848=CARTESIAN_POINT('Ctrl Pts',(-0.094379570415743,-0.25,0.00869613615398111));
#39849=CARTESIAN_POINT('Ctrl Pts',(-0.0502493781056048,-0.25,-1.73472347597681E-17));
#39850=CARTESIAN_POINT('',(-0.191381661893308,-0.168517237963823,3.46944695195361E-18));
#39851=CARTESIAN_POINT('Ctrl Pts',(-0.191381661893308,-0.168517237963823,
0.));
#39852=CARTESIAN_POINT('Ctrl Pts',(-0.169316565738238,-0.206735105578295,
0.00869613615398107));
#39853=CARTESIAN_POINT('Ctrl Pts',(-0.144337567297407,-0.25,0.0336751345948129));
#39854=CARTESIAN_POINT('Origin',(0.,0.,0.));
#39855=CARTESIAN_POINT('Origin',(0.,0.,0.0275));
#39856=CARTESIAN_POINT('',(0.144337567297406,-0.25,0.0336751345948129));
#39857=CARTESIAN_POINT('',(0.191381661893307,-0.168517237963823,3.46944695195361E-18));
#39858=CARTESIAN_POINT('Ctrl Pts',(0.144337567297406,-0.25,0.0336751345948129));
#39859=CARTESIAN_POINT('Ctrl Pts',(0.169316565738238,-0.206735105578296,
0.00869613615398108));
#39860=CARTESIAN_POINT('Ctrl Pts',(0.191381661893307,-0.168517237963823,
1.73472347597681E-17));
#39861=CARTESIAN_POINT('',(0.0502493781056045,-0.25,-1.73472347597681E-17));
#39862=CARTESIAN_POINT('Ctrl Pts',(0.0502493781056047,-0.25,-6.93889390390723E-18));
#39863=CARTESIAN_POINT('Ctrl Pts',(0.0943795704157429,-0.25,0.0086961361539811));
#39864=CARTESIAN_POINT('Ctrl Pts',(0.144337567297406,-0.25,0.0336751345948129));
#39865=CARTESIAN_POINT('Origin',(0.,0.,0.));
#39866=CARTESIAN_POINT('Origin',(0.,0.,0.0275));
#39867=CARTESIAN_POINT('',(0.241631039998912,-0.0814827620361769,1.04083408558608E-17));
#39868=CARTESIAN_POINT('',(0.288675134594813,0.,0.0336751345948129));
#39869=CARTESIAN_POINT('Ctrl Pts',(0.241631039998912,-0.0814827620361769,
2.08166817117217E-17));
#39870=CARTESIAN_POINT('Ctrl Pts',(0.263696136153981,-0.0432648944217041,
0.00869613615398126));
#39871=CARTESIAN_POINT('Ctrl Pts',(0.288675134594813,0.,0.0336751345948129));
#39872=CARTESIAN_POINT('',(0.241631039998912,0.0814827620361769,-6.93889390390723E-18));
#39873=CARTESIAN_POINT('Origin',(0.,0.,0.));
#39874=CARTESIAN_POINT('Ctrl Pts',(0.288675134594813,0.,0.0336751345948129));
#39875=CARTESIAN_POINT('Ctrl Pts',(0.263696136153981,0.0432648944217043,
0.0086961361539812));
#39876=CARTESIAN_POINT('Ctrl Pts',(0.241631039998912,0.0814827620361769,
3.12250225675825E-17));
#39877=CARTESIAN_POINT('Origin',(-0.144337567297407,-0.25,0.));
#39878=CARTESIAN_POINT('',(0.144337567297406,-0.25,0.966324865405187));
#39879=CARTESIAN_POINT('',(0.144337567297406,-0.25,0.));
#39880=CARTESIAN_POINT('',(0.0502493781056045,-0.25,1.));
#39881=CARTESIAN_POINT('Ctrl Pts',(0.144337567297406,-0.25,0.966324865405187));
#39882=CARTESIAN_POINT('Ctrl Pts',(0.0943795704157427,-0.25,0.991303863846019));
#39883=CARTESIAN_POINT('Ctrl Pts',(0.0502493781056045,-0.25,1.));
#39884=CARTESIAN_POINT('',(-0.0502493781056046,-0.25,1.));
#39885=CARTESIAN_POINT('',(-0.144337567297407,-0.25,1.));
#39886=CARTESIAN_POINT('',(-0.144337567297407,-0.25,0.966324865405187));
#39887=CARTESIAN_POINT('Ctrl Pts',(-0.0502493781056046,-0.25,1.));
#39888=CARTESIAN_POINT('Ctrl Pts',(-0.0943795704157429,-0.25,0.991303863846019));
#39889=CARTESIAN_POINT('Ctrl Pts',(-0.144337567297407,-0.25,0.966324865405187));
#39890=CARTESIAN_POINT('',(-0.144337567297407,-0.25,0.));
#39891=CARTESIAN_POINT('',(-0.144337567297407,-0.25,0.));
#39892=CARTESIAN_POINT('Origin',(-0.288675134594813,3.53525079574969E-17,
0.));
#39893=CARTESIAN_POINT('',(-0.191381661893308,-0.168517237963822,1.));
#39894=CARTESIAN_POINT('Ctrl Pts',(-0.144337567297407,-0.25,0.966324865405187));
#39895=CARTESIAN_POINT('Ctrl Pts',(-0.169316565738239,-0.206735105578295,
0.991303863846019));
#39896=CARTESIAN_POINT('Ctrl Pts',(-0.191381661893308,-0.168517237963823,
1.));
#39897=CARTESIAN_POINT('',(-0.241631039998912,-0.0814827620361775,1.));
#39898=CARTESIAN_POINT('',(-0.288675134594813,3.53525079574969E-17,1.));
#39899=CARTESIAN_POINT('',(-0.288675134594813,3.53525079574969E-17,0.966324865405187));
#39900=CARTESIAN_POINT('Ctrl Pts',(-0.241631039998912,-0.0814827620361772,
1.));
#39901=CARTESIAN_POINT('Ctrl Pts',(-0.263696136153981,-0.0432648944217047,
0.991303863846019));
#39902=CARTESIAN_POINT('Ctrl Pts',(-0.288675134594813,3.53525079574969E-17,
0.966324865405187));
#39903=CARTESIAN_POINT('',(-0.288675134594813,3.53525079574969E-17,0.));
#39904=CARTESIAN_POINT('',(-0.288675134594813,3.53525079574969E-17,0.));
#39905=CARTESIAN_POINT('Origin',(-0.144337567297406,0.25,0.));
#39906=CARTESIAN_POINT('',(-0.241631039998912,0.0814827620361772,1.));
#39907=CARTESIAN_POINT('Ctrl Pts',(-0.288675134594813,3.53525079574969E-17,
0.966324865405187));
#39908=CARTESIAN_POINT('Ctrl Pts',(-0.263696136153981,0.0432648944217045,
0.991303863846019));
#39909=CARTESIAN_POINT('Ctrl Pts',(-0.241631039998912,0.0814827620361772,
1.));
#39910=CARTESIAN_POINT('',(-0.191381661893307,0.168517237963823,1.));
#39911=CARTESIAN_POINT('',(-0.144337567297406,0.25,1.));
#39912=CARTESIAN_POINT('',(-0.144337567297406,0.25,0.966324865405187));
#39913=CARTESIAN_POINT('Ctrl Pts',(-0.191381661893307,0.168517237963823,
1.));
#39914=CARTESIAN_POINT('Ctrl Pts',(-0.169316565738238,0.206735105578295,
0.991303863846019));
#39915=CARTESIAN_POINT('Ctrl Pts',(-0.144337567297406,0.25,0.966324865405187));
#39916=CARTESIAN_POINT('',(-0.144337567297406,0.25,0.));
#39917=CARTESIAN_POINT('',(-0.144337567297406,0.25,0.));
#39918=CARTESIAN_POINT('Origin',(0.,0.,0.));
#39919=CARTESIAN_POINT('',(0.144337567297406,-0.25,0.));
#39920=CARTESIAN_POINT('',(0.144337567297406,0.25,0.));
#39921=CARTESIAN_POINT('',(0.288675134594813,0.,0.));
#39922=CARTESIAN_POINT('Origin',(0.144337567297406,0.25,0.));
#39923=CARTESIAN_POINT('',(-0.0502493781056043,0.25,1.));
#39924=CARTESIAN_POINT('Ctrl Pts',(-0.144337567297406,0.25,0.966324865405187));
#39925=CARTESIAN_POINT('Ctrl Pts',(-0.0943795704157428,0.25,0.991303863846019));
#39926=CARTESIAN_POINT('Ctrl Pts',(-0.0502493781056045,0.25,1.));
#39927=CARTESIAN_POINT('',(0.0502493781056044,0.25,1.));
#39928=CARTESIAN_POINT('',(0.144337567297406,0.25,1.));
#39929=CARTESIAN_POINT('',(0.144337567297406,0.25,0.966324865405187));
#39930=CARTESIAN_POINT('Ctrl Pts',(0.0502493781056046,0.25,1.));
#39931=CARTESIAN_POINT('Ctrl Pts',(0.0943795704157426,0.25,0.991303863846019));
#39932=CARTESIAN_POINT('Ctrl Pts',(0.144337567297406,0.25,0.966324865405187));
#39933=CARTESIAN_POINT('',(0.144337567297406,0.25,0.));
#39934=CARTESIAN_POINT('Origin',(0.,0.,0.9725));
#39935=CARTESIAN_POINT('',(0.241631039998912,0.0814827620361773,1.));
#39936=CARTESIAN_POINT('',(0.288675134594813,0.,0.966324865405187));
#39937=CARTESIAN_POINT('Ctrl Pts',(0.241631039998912,0.0814827620361773,
1.));
#39938=CARTESIAN_POINT('Ctrl Pts',(0.263696136153981,0.0432648944217048,
0.991303863846019));
#39939=CARTESIAN_POINT('Ctrl Pts',(0.288675134594813,0.,0.966324865405187));
#39940=CARTESIAN_POINT('',(0.241631039998912,-0.0814827620361771,1.));
#39941=CARTESIAN_POINT('Origin',(0.,0.,1.));
#39942=CARTESIAN_POINT('Ctrl Pts',(0.288675134594813,0.,0.966324865405187));
#39943=CARTESIAN_POINT('Ctrl Pts',(0.263696136153981,-0.0432648944217043,
0.991303863846019));
#39944=CARTESIAN_POINT('Ctrl Pts',(0.241631039998912,-0.0814827620361776,
1.));
#39945=CARTESIAN_POINT('Origin',(0.,0.,0.9725));
#39946=CARTESIAN_POINT('',(0.191381661893308,0.168517237963823,1.));
#39947=CARTESIAN_POINT('Origin',(0.,0.,1.));
#39948=CARTESIAN_POINT('Ctrl Pts',(0.144337567297406,0.25,0.966324865405187));
#39949=CARTESIAN_POINT('Ctrl Pts',(0.169316565738239,0.206735105578295,
0.991303863846019));
#39950=CARTESIAN_POINT('Ctrl Pts',(0.191381661893308,0.168517237963823,
1.));
#39951=CARTESIAN_POINT('Origin',(0.,0.,0.9725));
#39952=CARTESIAN_POINT('Origin',(0.,0.,1.));
#39953=CARTESIAN_POINT('Origin',(0.,0.,0.9725));
#39954=CARTESIAN_POINT('Origin',(0.,0.,1.));
#39955=CARTESIAN_POINT('Origin',(0.,0.,0.9725));
#39956=CARTESIAN_POINT('Origin',(0.,0.,1.));
#39957=CARTESIAN_POINT('Origin',(0.,0.,0.9725));
#39958=CARTESIAN_POINT('',(0.191381661893308,-0.168517237963823,1.));
#39959=CARTESIAN_POINT('Ctrl Pts',(0.191381661893308,-0.168517237963822,
1.));
#39960=CARTESIAN_POINT('Ctrl Pts',(0.169316565738238,-0.206735105578296,
0.991303863846019));
#39961=CARTESIAN_POINT('Ctrl Pts',(0.144337567297406,-0.25,0.966324865405187));
#39962=CARTESIAN_POINT('Origin',(0.,0.,1.));
#39963=CARTESIAN_POINT('Origin',(0.144337567297406,-0.25,0.));
#39964=CARTESIAN_POINT('',(0.288675134594813,0.,0.));
#39965=CARTESIAN_POINT('',(0.144337567297406,-0.25,1.));
#39966=CARTESIAN_POINT('Origin',(0.105,0.,-0.4));
#39967=CARTESIAN_POINT('',(-0.105,-1.28587913910472E-17,-0.4));
#39968=CARTESIAN_POINT('Origin',(0.,0.,-0.4));
#39969=CARTESIAN_POINT('Origin',(0.,0.,-0.39));
#39970=CARTESIAN_POINT('',(-0.115,-1.40834381901946E-17,-0.39));
#39971=CARTESIAN_POINT('Origin',(0.288675134594813,0.,0.));
#39972=CARTESIAN_POINT('',(0.288675134594813,0.,1.));
#39973=CARTESIAN_POINT('Origin',(0.,0.,1.));
#54974=UNCERTAINTY_MEASURE_WITH_UNIT(LENGTH_MEASURE(0.001),#55003,
'DISTANCE_ACCURACY_VALUE',
'Maximum model space distance between geometric entities at asserted c
onnectivities');
#54980=UNCERTAINTY_MEASURE_WITH_UNIT(LENGTH_MEASURE(0.001),#55003,
'DISTANCE_ACCURACY_VALUE',
'Maximum model space distance between geometric entities at asserted c
onnectivities');
#54996=(
GEOMETRIC_REPRESENTATION_CONTEXT(3)
GLOBAL_UNCERTAINTY_ASSIGNED_CONTEXT((#54974))
GLOBAL_UNIT_ASSIGNED_CONTEXT((#55003,#55005,#55006))
REPRESENTATION_CONTEXT('','3D')
);
#55002=(
GEOMETRIC_REPRESENTATION_CONTEXT(3)
GLOBAL_UNCERTAINTY_ASSIGNED_CONTEXT((#54980))
GLOBAL_UNIT_ASSIGNED_CONTEXT((#55003,#55005,#55006))
REPRESENTATION_CONTEXT('','3D')
);
#55003=(
LENGTH_UNIT()
NAMED_UNIT(*)
SI_UNIT(.CENTI.,.METRE.)
);
#55005=(
NAMED_UNIT(*)
PLANE_ANGLE_UNIT()
SI_UNIT($,.RADIAN.)
);
#55006=(
NAMED_UNIT(*)
SI_UNIT($,.STERADIAN.)
SOLID_ANGLE_UNIT()
);
#55022=SHAPE_DEFINITION_REPRESENTATION(#55043,#55118);
#55043=PRODUCT_DEFINITION_SHAPE('',$,#55140);
#55118=SHAPE_REPRESENTATION('',(#26185),#54996);
#55124=PRODUCT_DEFINITION_CONTEXT('part definition',#55189,'design');
#55140=PRODUCT_DEFINITION('2026-10-18-23-36-48-728',
'14_Hex_Standoff_M2.5_AF5x10_Male-Female',#55161,#55124);
#55161=PRODUCT_DEFINITION_FORMATION('',$,#55206);
#55189=APPLICATION_CONTEXT(
'Core Data for Automotive Mechanical Design Process');
#55190=PRODUCT_CONTEXT('part definition',#55189,'mechanical');
#55206=PRODUCT('2026-10-18-23-36-48-728',
'14_Hex_Standoff_M2.5_AF5x10_Male-Female',$,(#55190));
#55373=COLOUR_RGB('Sky Blue',0.24,0.69,0.87);
#55374=FILL_AREA_STYLE_COLOUR('',#55373);
#55375=FILL_AREA_STYLE('',(#55374));
#55376=SURFACE_STYLE_FILL_AREA(#55375);
#55377=SURFACE_SIDE_STYLE('',(#55376));
#55378=SURFACE_STYLE_USAGE(.BOTH.,#55377);
#55379=PRESENTATION_STYLE_ASSIGNMENT((#55378));
ENDSEC;
END-ISO-10303-21;
